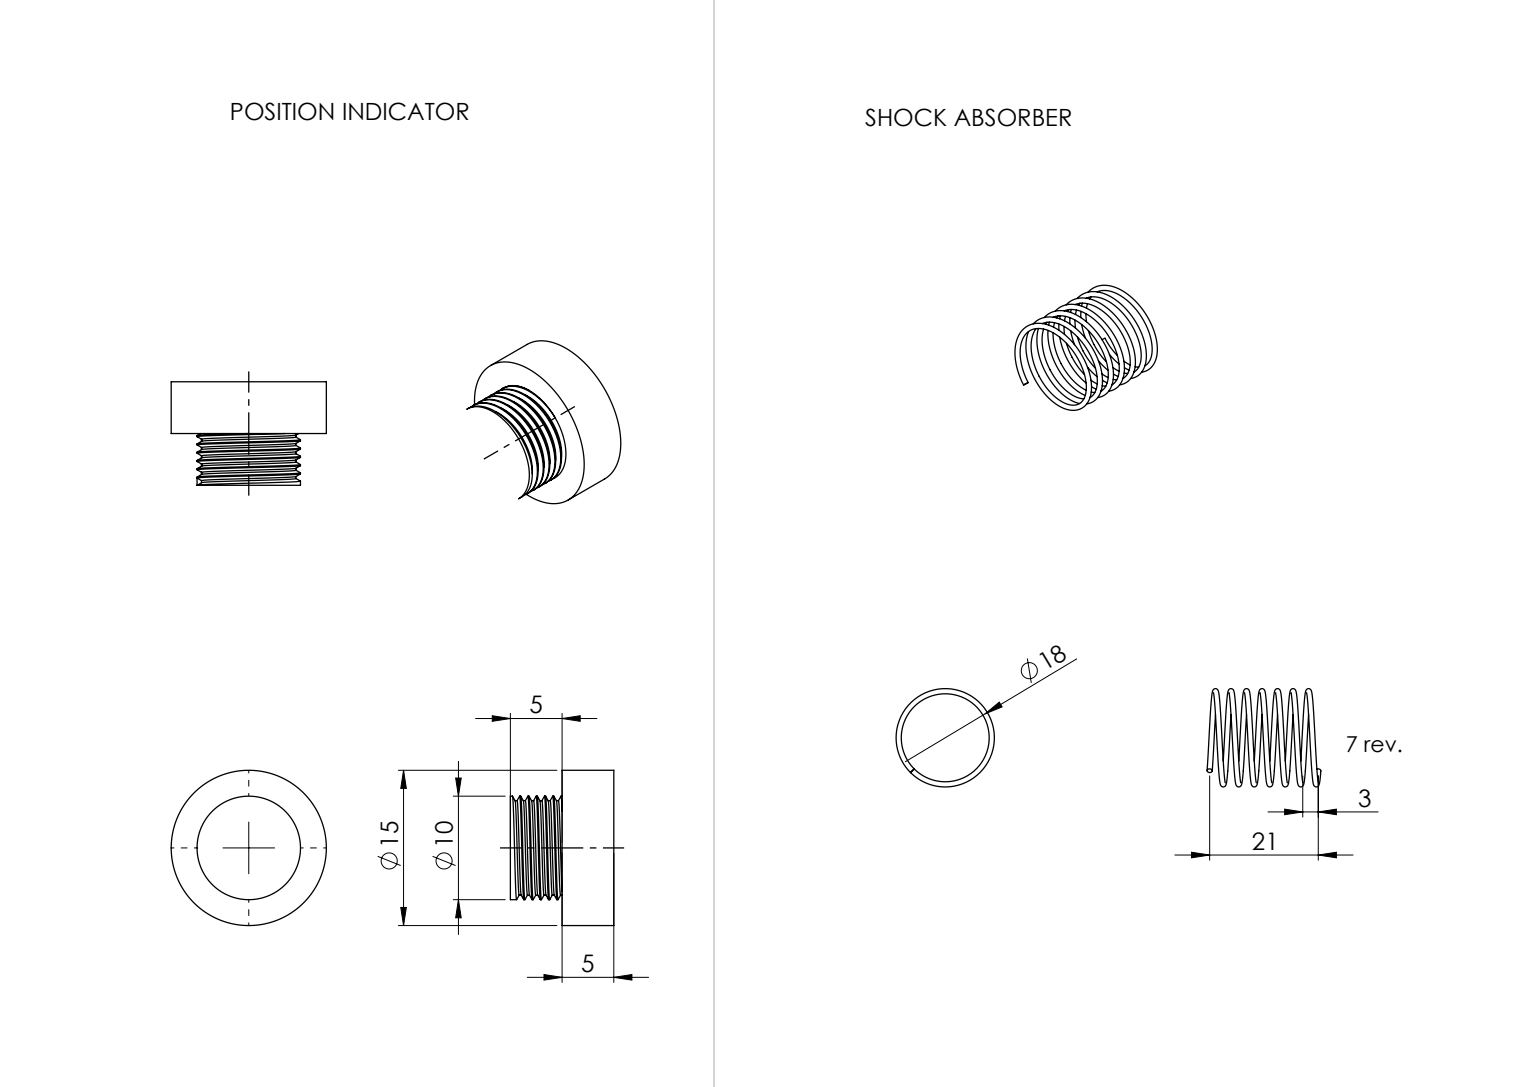
ISO-10303-21;
HEADER;
FILE_DESCRIPTION (('STEP AP214'),
    '1' );
FILE_NAME ('shock absorber.step',
    '2026-09-29T11:11:29',
    ( '' ),
    ( '' ),
    'SwSTEP 2.0',
    'SolidWorks 2026',
    '' );
FILE_SCHEMA (( 'AUTOMOTIVE_DESIGN' ));
ENDSEC;

DATA;
#6=CARTESIAN_POINT ( 'NONE',  ( -39.38303923565386100, -41.70000000000000995, -1.486127417882099788 ) ) ;
#7=CARTESIAN_POINT ( 'NONE',  ( -22.03669253526174998, -31.34999999999999787, 4.057507815433014642 ) ) ;
#11=CARTESIAN_POINT ( 'NONE',  ( -21.55948914237271907, -43.89859572486944472, -4.360112732550413206 ) ) ;
#17=CARTESIAN_POINT ( 'NONE',  ( -28.67030704715798350, -46.80000000000001137, 8.395350895058669494 ) ) ;
#18=CARTESIAN_POINT ( 'NONE',  ( -31.50758917197619979, -41.94859572486944188, 9.874625247442176956 ) ) ;
#19=CARTESIAN_POINT ( 'NONE',  ( -22.89739904353894318, -38.75140427513058228, -7.023824353025938549 ) ) ;
#23=CARTESIAN_POINT ( 'NONE',  ( -21.12512167993187973, -48.35140427513057659, 4.584493831696868860 ) ) ;
#30=CARTESIAN_POINT ( 'NONE',  ( -22.03669253526174998, -49.35000000000000853, 4.057507815433014642 ) ) ;
#31=CARTESIAN_POINT ( 'NONE',  ( -23.28248557872775137, -37.50000000000000711, 6.717514421272141156 ) ) ;
#36=CARTESIAN_POINT ( 'NONE',  ( -34.53486167607238144, -42.15000000000001279, -8.900167166472096270 ) ) ;
#40=CARTESIAN_POINT ( 'NONE',  ( -28.54686042191934092, -41.45140427513058512, -8.818680382772479120 ) ) ;
#43=CARTESIAN_POINT ( 'NONE',  ( -23.68028341417693738, -42.75000000000000711, -6.319716585823200283 ) ) ;
#50=CARTESIAN_POINT ( 'NONE',  ( -21.09983283352784156, -49.35000000000000853, 4.534861676072186043 ) ) ;
#51=CARTESIAN_POINT ( 'NONE',  ( -21.17260567462091458, -31.05000000000000782, -1.398121909749242331 ) ) ;
#55=CARTESIAN_POINT ( 'NONE',  ( -23.24502507771338600, -44.49859572486944614, 6.680053920257780220 ) ) ;
#57=CARTESIAN_POINT ( 'NONE',  ( -21.09983283352783801, -34.35000000000000853, 4.534861676072186043 ) ) ;
#61=CARTESIAN_POINT ( 'NONE',  ( -34.10713997105786888, -31.14859572486944828, -7.938018618334151455 ) ) ;
#62=CARTESIAN_POINT ( 'NONE',  ( -25.73429323749904185, -40.59859572486944757, -8.488613101951701267 ) ) ;
#63=CARTESIAN_POINT ( 'NONE',  ( -31.61762450863942320, -45.95140427513058512, 9.857197362228843573 ) ) ;
#64=ORIENTED_EDGE ( 'NONE', *, *, #7792, .F. ) ;
#66=CARTESIAN_POINT ( 'NONE',  ( -22.89739904353894318, -41.75140427513057517, -7.023824353025938549 ) ) ;
#72=CARTESIAN_POINT ( 'NONE',  ( -31.38201786482021305, -34.29859572486943620, -8.387063443159975762 ) ) ;
#73=CARTESIAN_POINT ( 'NONE',  ( -39.86591130483550671, -32.55000000000000426, 1.562606840307984468 ) ) ;
#84=CARTESIAN_POINT ( 'NONE',  ( -31.45313957808072303, -39.95140427513058512, 8.818680382772479120 ) ) ;
#91=CARTESIAN_POINT ( 'NONE',  ( -22.03669253526174998, -43.35000000000000853, 4.057507815433014642 ) ) ;
#97=CARTESIAN_POINT ( 'NONE',  ( -25.46513832392765408, -46.65000000000001279, 8.900167166472096270 ) ) ;
#98=CARTESIAN_POINT ( 'NONE',  ( -34.05750781543318340, -33.15000000000001279, -7.963307464738195840 ) ) ;
#103=CARTESIAN_POINT ( 'NONE',  ( -25.73429323749904185, -43.59859572486944046, -8.488613101951701267 ) ) ;
#105=CARTESIAN_POINT ( 'NONE',  ( -23.28248557872775137, -34.50000000000000000, 6.717514421272141156 ) ) ;
#106=EDGE_LOOP ( 'NONE', ( #3791, #8082, #1167, #64 ) ) ;
#109=CARTESIAN_POINT ( 'NONE',  ( -25.94249218456686279, -46.65000000000001279, 7.963307464738195840 ) ) ;
#110=CARTESIAN_POINT ( 'NONE',  ( -31.53845232986046554, -43.29859572486943620, -9.374751783755117529 ) ) ;
#111=CARTESIAN_POINT ( 'NONE',  ( -36.68005392025794009, -41.00140427513057517, -6.754974922286504757 ) ) ;
#115=CARTESIAN_POINT ( 'NONE',  ( -23.28248557872775137, -31.50000000000000711, 6.717514421272141156 ) ) ;
#121=CARTESIAN_POINT ( 'NONE',  ( -33.85891924778610473, -50.10000000000000853, 7.573555455601171715 ) ) ;
#122=CARTESIAN_POINT ( 'NONE',  ( -25.46513832392765408, -31.65000000000000568, 8.900167166472096270 ) ) ;
#124=CARTESIAN_POINT ( 'NONE',  ( -20.13408869516453947, -46.05000000000001137, -1.562606840307983136 ) ) ;
#131=CARTESIAN_POINT ( 'NONE',  ( -38.83610826798580717, -46.55140427513058654, 1.343104241417631073 ) ) ;
#134=CARTESIAN_POINT ( 'NONE',  ( -31.32969295284206979, -48.30000000000001137, -8.395350895058669494 ) ) ;
#142=CARTESIAN_POINT ( 'NONE',  ( -25.94249218456686279, -34.64999999999998437, 7.963307464738195840 ) ) ;
#146=CARTESIAN_POINT ( 'NONE',  ( -34.58449383169706692, -46.14859572486944472, -8.874878320068054549 ) ) ;
#148=CARTESIAN_POINT ( 'NONE',  ( -20.61696076434619584, -34.20000000000000995, 1.486127417882100676 ) ) ;
#153=CARTESIAN_POINT ( 'NONE',  ( -21.59636165304264921, -38.19859572486942767, 1.277368040863740228 ) ) ;
#155=CARTESIAN_POINT ( 'NONE',  ( -21.07454398712378918, -44.34859572486944046, 4.485229520447505003 ) ) ;
#156=CARTESIAN_POINT ( 'NONE',  ( -39.37475178375516549, -43.70140427513058512, -1.538452329860249712 ) ) ;
#167=CARTESIAN_POINT ( 'NONE',  ( -38.81868038277247734, -36.54859572486943620, 1.453139578080855365 ) ) ;
#168=CARTESIAN_POINT ( 'NONE',  ( -36.71751442127229836, -30.00000000000000711, -6.717514421272142044 ) ) ;
#170=CARTESIAN_POINT ( 'NONE',  ( -25.68709025247441602, -48.60000000000000142, -8.464561979789547053 ) ) ;
#178=CARTESIAN_POINT ( 'NONE',  ( -23.64089511245930098, -44.75140427513058228, -6.280328284105564762 ) ) ;
#182=CARTESIAN_POINT ( 'NONE',  ( -23.68028341417693738, -48.75000000000000711, -6.319716585823200283 ) ) ;
#185=CARTESIAN_POINT ( 'NONE',  ( -21.60464910494133406, -37.20000000000000284, 1.329692952841886155 ) ) ;
#190=CARTESIAN_POINT ( 'NONE',  ( -38.44051085762733777, -45.39859572486944472, 4.360112732550414982 ) ) ;
#192=CARTESIAN_POINT ( 'NONE',  ( -34.31290974752564438, -32.10000000000000142, 8.464561979789547053 ) ) ;
#197=CARTESIAN_POINT ( 'NONE',  ( -26.18828373723858149, -43.59859572486944046, -7.597606577763319713 ) ) ;
#198=CARTESIAN_POINT ( 'NONE',  ( -25.68709025247441602, -30.60000000000000142, -8.464561979789547053 ) ) ;
#199=CARTESIAN_POINT ( 'NONE',  ( -38.83610826798580717, -31.55140427513057588, 1.343104241417631073 ) ) ;
#208=CARTESIAN_POINT ( 'NONE',  ( -31.38201786482021305, -46.29859572486944330, -8.387063443159975762 ) ) ;
#209=CARTESIAN_POINT ( 'NONE',  ( -34.31290974752564438, -41.10000000000000142, 8.464561979789547053 ) ) ;
#211=CARTESIAN_POINT ( 'NONE',  ( -36.71751442127229836, -45.00000000000000711, -6.717514421272142044 ) ) ;
#219=CARTESIAN_POINT ( 'NONE',  ( -37.93801861833426159, -40.85140427513057659, -4.107139971057695682 ) ) ;
#223=CARTESIAN_POINT ( 'NONE',  ( -28.67030704715798350, -46.80000000000001137, 8.395350895058669494 ) ) ;
#227=CARTESIAN_POINT ( 'NONE',  ( -23.68028341417693738, -42.75000000000001421, -6.319716585823198507 ) ) ;
#230=CARTESIAN_POINT ( 'NONE',  ( -34.53486167607238144, -33.15000000000001279, -8.900167166472096270 ) ) ;
#232=CARTESIAN_POINT ( 'NONE',  ( -21.53543802021056663, -36.90000000000000568, -4.312909747525783821 ) ) ;
#237=CARTESIAN_POINT ( 'NONE',  ( -22.45049566656107842, -40.89859572486943762, -3.906122232810846917 ) ) ;
#238=CARTESIAN_POINT ( 'NONE',  ( -21.53543802021056663, -30.90000000000000924, -4.312909747525783821 ) ) ;
#239=CARTESIAN_POINT ( 'NONE',  ( -36.68005392025794009, -47.00140427513058938, -6.754974922286504757 ) ) ;
#251=CARTESIAN_POINT ( 'NONE',  ( -37.98859631114233792, -39.84859572486944046, -4.007875659808334490 ) ) ;
#252=CARTESIAN_POINT ( 'NONE',  ( -25.46513832392765408, -43.64999999999999147, 8.900167166472096270 ) ) ;
#254=CARTESIAN_POINT ( 'NONE',  ( -34.48522952044771017, -29.15140427513058441, -8.925456012876139766 ) ) ;
#261=CARTESIAN_POINT ( 'NONE',  ( -25.94249218456686279, -34.64999999999998437, 7.963307464738195840 ) ) ;
#266=CARTESIAN_POINT ( 'NONE',  ( -36.01040764008574513, -51.00000000000000711, -6.010407640085605685 ) ) ;
#270=CARTESIAN_POINT ( 'NONE',  ( -22.42644454439892598, -36.90000000000000568, -3.858919247786222861 ) ) ;
#274=CARTESIAN_POINT ( 'NONE',  ( -37.06321265474346660, -32.25000000000000711, 7.063212654743582952 ) ) ;
#277=CARTESIAN_POINT ( 'NONE',  ( -23.28248557872775137, -43.50000000000001421, 6.717514421272141156 ) ) ;
#278=SURFACE_STYLE_FILL_AREA ( #8401 ) ;
#282=VERTEX_POINT ( 'NONE', #3656 ) ;
#283=CARTESIAN_POINT ( 'NONE',  ( -33.81171626276147890, -39.09859572486944046, 7.597606577763319713 ) ) ;
#284=CARTESIAN_POINT ( 'NONE',  ( -31.50758917197619979, -50.94859572486944899, 9.874625247442176956 ) ) ;
#285=CARTESIAN_POINT ( 'NONE',  ( -26.09387776718931917, -29.60140427513057659, -7.549504333439021941 ) ) ;
#294=CARTESIAN_POINT ( 'NONE',  ( -23.71967171589458445, -40.74859572486943904, -6.359104887540838469 ) ) ;
#295=CARTESIAN_POINT ( 'NONE',  ( -38.46456197978948666, -41.40000000000000568, 4.312909747525784709 ) ) ;
#298=CARTESIAN_POINT ( 'NONE',  ( -21.12512167993187973, -30.35140427513058015, 4.584493831696868860 ) ) ;
#306=CARTESIAN_POINT ( 'NONE',  ( -33.85891924778610473, -35.10000000000000853, 7.573555455601171715 ) ) ;
#310=CIRCLE ( 'NONE', #7910, 0.5000000000000001110 ) ;
#314=CARTESIAN_POINT ( 'NONE',  ( -38.39535089505872634, -35.70000000000000995, -1.329692952841885267 ) ) ;
#318=CARTESIAN_POINT ( 'NONE',  ( -25.46513832392765408, -37.65000000000000568, 8.900167166472096270 ) ) ;
#320=CARTESIAN_POINT ( 'NONE',  ( -37.06321265474346660, -44.25000000000000000, 7.063212654743582952 ) ) ;
#321=( NAMED_UNIT ( * ) PLANE_ANGLE_UNIT ( ) SI_UNIT ( $, .RADIAN. ) );
#324=CARTESIAN_POINT ( 'NONE',  ( -34.10713997105786888, -43.14859572486943762, -7.938018618334151455 ) ) ;
#325=CARTESIAN_POINT ( 'NONE',  ( -28.49241082802385350, -49.44859572486943478, -9.874625247442173404 ) ) ;
#326=CARTESIAN_POINT ( 'NONE',  ( -37.59760657776328685, -31.40140427513058086, 3.811716262761598362 ) ) ;
#329=CARTESIAN_POINT ( 'NONE',  ( -21.09983283352784156, -40.35000000000000142, 4.534861676072186043 ) ) ;
#334=CARTESIAN_POINT ( 'NONE',  ( -22.01140368885771892, -38.34859572486944046, 4.007875659808335378 ) ) ;
#336=CARTESIAN_POINT ( 'NONE',  ( -22.93678734525658314, -42.75000000000001421, -7.063212654743582952 ) ) ;
#338=CARTESIAN_POINT ( 'NONE',  ( -25.51477047955235378, -39.65140427513058086, 8.925456012876139766 ) ) ;
#345=CARTESIAN_POINT ( 'NONE',  ( -26.14108075221394856, -30.60000000000000142, -7.573555455601170827 ) ) ;
#352=CARTESIAN_POINT ( 'NONE',  ( -36.31971658582311591, -44.25000000000000000, 6.319716585823199395 ) ) ;
#357=CARTESIAN_POINT ( 'NONE',  ( -21.53543802021056663, -36.90000000000000568, -4.312909747525783821 ) ) ;
#359=CARTESIAN_POINT ( 'NONE',  ( -25.68709025247441602, -36.60000000000000853, -8.464561979789547053 ) ) ;
#361=CARTESIAN_POINT ( 'NONE',  ( -36.04786814110010340, -51.99859572486943193, -5.972947139071243861 ) ) ;
#362=CARTESIAN_POINT ( 'NONE',  ( -20.61696076434619584, -31.20000000000000639, 1.486127417882100676 ) ) ;
#363=CARTESIAN_POINT ( 'NONE',  ( -23.64089511245930098, -32.75140427513057517, -6.280328284105564762 ) ) ;
#367=CARTESIAN_POINT ( 'NONE',  ( -21.53543802021056663, -33.90000000000000568, -4.312909747525783821 ) ) ;
#369=CARTESIAN_POINT ( 'NONE',  ( -36.01040764008574513, -30.00000000000000711, -6.010407640085605685 ) ) ;
#374=CARTESIAN_POINT ( 'NONE',  ( -37.54950433343896776, -45.39859572486944472, 3.906122232810848249 ) ) ;
#375=CARTESIAN_POINT ( 'NONE',  ( -31.48612741788231517, -45.30000000000000426, -9.383039235653804155 ) ) ;
#377=ORIENTED_EDGE ( 'NONE', *, *, #4137, .F. ) ;
#378=CARTESIAN_POINT ( 'NONE',  ( -36.68005392025794009, -32.00140427513057517, -6.754974922286504757 ) ) ;
#386=CARTESIAN_POINT ( 'NONE',  ( -33.90612223281073057, -49.10140427513058370, 7.549504333439023718 ) ) ;
#397=CARTESIAN_POINT ( 'NONE',  ( -20.13408869516454303, -43.04999999999999716, -1.562606840307982692 ) ) ;
#399=CARTESIAN_POINT ( 'NONE',  ( -28.49241082802385350, -31.44859572486944188, -9.874625247442173404 ) ) ;
#400=CARTESIAN_POINT ( 'NONE',  ( -25.46513832392765408, -40.65000000000000568, 8.900167166472096270 ) ) ;
#401=CARTESIAN_POINT ( 'NONE',  ( -23.64089511245930098, -35.75140427513057517, -6.280328284105564762 ) ) ;
#404=CARTESIAN_POINT ( 'NONE',  ( -20.13408869516453947, -34.04999999999998295, -1.562606840307983136 ) ) ;
#411=CARTESIAN_POINT ( 'NONE',  ( -37.98859631114233792, -51.84859572486944757, -4.007875659808334490 ) ) ;
#412=CARTESIAN_POINT ( 'NONE',  ( -25.46513832392765408, -49.64999999999999147, 8.900167166472096270 ) ) ;
#415=CARTESIAN_POINT ( 'NONE',  ( -21.12512167993187973, -39.35140427513057659, 4.584493831696868860 ) ) ;
#416=CIRCLE ( 'NONE', #3111, 0.5000000000000001110 ) ;
#422=CARTESIAN_POINT ( 'NONE',  ( -22.42644454439892598, -36.90000000000000568, -3.858919247786222861 ) ) ;
#435=CARTESIAN_POINT ( 'NONE',  ( -21.09983283352783801, -46.34999999999999432, 4.534861676072186043 ) ) ;
#437=CARTESIAN_POINT ( 'NONE',  ( -38.81868038277247734, -45.54859572486944330, 1.453139578080855365 ) ) ;
#438=CARTESIAN_POINT ( 'NONE',  ( -21.53543802021056663, -36.90000000000000568, -4.312909747525783821 ) ) ;
#440=CARTESIAN_POINT ( 'NONE',  ( -37.59760657776328685, -40.40140427513058086, 3.811716262761598362 ) ) ;
#444=CARTESIAN_POINT ( 'NONE',  ( -38.92545601287626056, -36.84859572486944046, -4.485229520447501450 ) ) ;
#445=CARTESIAN_POINT ( 'NONE',  ( -31.48612741788231517, -36.30000000000000426, -9.383039235653804155 ) ) ;
#452=CARTESIAN_POINT ( 'NONE',  ( -31.38201786482021305, -49.29859572486945041, -8.387063443159975762 ) ) ;
#453=CARTESIAN_POINT ( 'NONE',  ( -21.12512167993187973, -33.35140427513057659, 4.584493831696868860 ) ) ;
#457=CARTESIAN_POINT ( 'NONE',  ( -21.51138689804841420, -35.90140427513058086, -4.265706762501151772 ) ) ;
#464=CARTESIAN_POINT ( 'NONE',  ( -37.96330746473829976, -38.85000000000001563, -4.057507815433013754 ) ) ;
#470=CARTESIAN_POINT ( 'NONE',  ( -24.02705286092866643, -33.50140427513058228, 6.047868141099968398 ) ) ;
#473=CARTESIAN_POINT ( 'NONE',  ( -23.68028341417693738, -36.75000000000000711, -6.319716585823200283 ) ) ;
#475=CARTESIAN_POINT ( 'NONE',  ( -37.06321265474346660, -47.25000000000000711, 7.063212654743582952 ) ) ;
#478=CARTESIAN_POINT ( 'NONE',  ( -26.18828373723858149, -46.59859572486944046, -7.597606577763319713 ) ) ;
#479=CARTESIAN_POINT ( 'NONE',  ( -39.86591130483550671, -38.54999999999999716, 1.562606840307984468 ) ) ;
#480=CARTESIAN_POINT ( 'NONE',  ( -33.90612223281073057, -40.10140427513057659, 7.549504333439023718 ) ) ;
#484=CARTESIAN_POINT ( 'NONE',  ( -21.55948914237271907, -40.89859572486943762, -4.360112732550413206 ) ) ;
#485=CARTESIAN_POINT ( 'NONE',  ( -38.46456197978948666, -35.40000000000000568, 4.312909747525784709 ) ) ;
#493=CARTESIAN_POINT ( 'NONE',  ( -34.26570676250101855, -33.09859572486943335, 8.488613101951703044 ) ) ;
#494=CARTESIAN_POINT ( 'NONE',  ( -28.56619749409589204, -33.80140427513056522, 9.391326687552490782 ) ) ;
#496=AXIS2_PLACEMENT_3D ( 'NONE', #718, #6149, #4079 ) ;
#499=CARTESIAN_POINT ( 'NONE',  ( -25.63988726744978663, -38.60140427513057659, -8.440510857627391061 ) ) ;
#507=CARTESIAN_POINT ( 'NONE',  ( -21.60464910494133406, -40.20000000000000995, 1.329692952841886155 ) ) ;
#513=CARTESIAN_POINT ( 'NONE',  ( -39.38303923565386100, -35.70000000000000995, -1.486127417882099788 ) ) ;
#516=CARTESIAN_POINT ( 'NONE',  ( -34.00787565980851213, -32.15140427513058086, -7.988596311142238449 ) ) ;
#519=CARTESIAN_POINT ( 'NONE',  ( -38.82739432537914581, -38.55000000000000426, 1.398121909749243663 ) ) ;
#521=CARTESIAN_POINT ( 'NONE',  ( -21.53543802021056663, -48.90000000000000568, -4.312909747525783821 ) ) ;
#524=CARTESIAN_POINT ( 'NONE',  ( -37.54950433343896776, -48.39859572486944472, 3.906122232810848249 ) ) ;
#525=CARTESIAN_POINT ( 'NONE',  ( -39.38303923565386100, -35.70000000000000995, -1.486127417882099788 ) ) ;
#526=CARTESIAN_POINT ( 'NONE',  ( -35.97294713907137975, -35.00140427513057517, -6.047868141099968398 ) ) ;
#530=CARTESIAN_POINT ( 'NONE',  ( -31.50758917197619979, -41.94859572486944188, 9.874625247442176956 ) ) ;
#531=CARTESIAN_POINT ( 'NONE',  ( -20.61696076434619584, -43.20000000000000995, 1.486127417882100676 ) ) ;
#539=CARTESIAN_POINT ( 'NONE',  ( -21.59636165304264921, -47.19859572486943478, 1.277368040863740228 ) ) ;
#540=CARTESIAN_POINT ( 'NONE',  ( -39.87462524744216807, -34.55140427513057233, 1.507589171976367215 ) ) ;
#543=CARTESIAN_POINT ( 'NONE',  ( -28.38237549136062654, -44.45140427513058512, -9.857197362228843573 ) ) ;
#551=CARTESIAN_POINT ( 'NONE',  ( -38.39535089505872634, -44.70000000000000284, -1.329692952841885267 ) ) ;
#555=CARTESIAN_POINT ( 'NONE',  ( -22.93678734525658314, -39.74999999999999289, -7.063212654743582952 ) ) ;
#559=CARTESIAN_POINT ( 'NONE',  ( -37.93801861833426159, -37.85140427513057659, -4.107139971057695682 ) ) ;
#562=CARTESIAN_POINT ( 'NONE',  ( -34.05750781543319050, -39.14999999999999858, -7.963307464738194952 ) ) ;
#565=CARTESIAN_POINT ( 'NONE',  ( -39.86591130483550671, -50.55000000000001137, 1.562606840307984690 ) ) ;
#569=CARTESIAN_POINT ( 'NONE',  ( -36.71751442127229836, -39.00000000000000711, -6.717514421272142044 ) ) ;
#570=CARTESIAN_POINT ( 'NONE',  ( -34.00787565980851213, -38.15140427513058086, -7.988596311142238449 ) ) ;
#573=CARTESIAN_POINT ( 'NONE',  ( -25.41550616830297571, -32.64859572486943762, 8.874878320068054549 ) ) ;
#574=CARTESIAN_POINT ( 'NONE',  ( -31.50758917197619979, -32.94859572486944188, 9.874625247442176956 ) ) ;
#582=CARTESIAN_POINT ( 'NONE',  ( -36.01040764008574513, -48.00000000000000711, -6.010407640085605685 ) ) ;
#583=CARTESIAN_POINT ( 'NONE',  ( -23.24502507771338600, -32.49859572486943904, 6.680053920257780220 ) ) ;
#584=CARTESIAN_POINT ( 'NONE',  ( -20.62524821624488069, -36.20140427513057091, 1.538452329860250378 ) ) ;
#588=CARTESIAN_POINT ( 'NONE',  ( -20.12537475255788522, -42.05140427513057944, -1.507589171976365439 ) ) ;
#596=CARTESIAN_POINT ( 'NONE',  ( -31.39812190974910422, -43.95000000000000284, 8.827394325379140483 ) ) ;
#601=CARTESIAN_POINT ( 'NONE',  ( -31.48612741788231517, -42.30000000000000426, -9.383039235653804155 ) ) ;
#604=CARTESIAN_POINT ( 'NONE',  ( -22.06198138166579170, -36.35140427513057659, 4.107139971057695682 ) ) ;
#609=CARTESIAN_POINT ( 'NONE',  ( -36.31971658582311591, -38.25000000000000711, 6.319716585823200283 ) ) ;
#611=CARTESIAN_POINT ( 'NONE',  ( -28.43739315969223824, -48.45000000000000284, -9.865911304835512041 ) ) ;
#616=CARTESIAN_POINT ( 'NONE',  ( -31.48612741788231517, -42.30000000000000426, -9.383039235653804155 ) ) ;
#617=CARTESIAN_POINT ( 'NONE',  ( -26.09387776718931917, -44.60140427513058370, -7.549504333439021941 ) ) ;
#621=CARTESIAN_POINT ( 'NONE',  ( -34.58449383169706692, -40.14859572486943762, -8.874878320068054549 ) ) ;
#628=CARTESIAN_POINT ( 'NONE',  ( -25.94249218456686279, -49.64999999999999147, 7.963307464738195840 ) ) ;
#630=CARTESIAN_POINT ( 'NONE',  ( -39.39132668755255651, -39.69859572486944188, -1.433802505903950308 ) ) ;
#631=CARTESIAN_POINT ( 'NONE',  ( -25.63988726744978663, -44.60140427513058370, -8.440510857627391061 ) ) ;
#635=CARTESIAN_POINT ( 'NONE',  ( -37.10260095646111012, -46.25140427513058228, 7.023824353025939438 ) ) ;
#643=CARTESIAN_POINT ( 'NONE',  ( -31.39812190974910422, -46.94999999999998863, 8.827394325379140483 ) ) ;
#649=CARTESIAN_POINT ( 'NONE',  ( -20.13408869516453947, -40.05000000000001137, -1.562606840307983136 ) ) ;
#652=CARTESIAN_POINT ( 'NONE',  ( -23.64089511245930098, -32.75140427513057517, -6.280328284105564762 ) ) ;
#657=CARTESIAN_POINT ( 'NONE',  ( -26.14108075221394856, -39.60000000000000853, -7.573555455601170827 ) ) ;
#664=CARTESIAN_POINT ( 'NONE',  ( -20.61696076434619584, -43.20000000000000995, 1.486127417882100676 ) ) ;
#665=CARTESIAN_POINT ( 'NONE',  ( -31.27736804086391942, -44.30140427513057944, -8.403638346957361449 ) ) ;
#669=CARTESIAN_POINT ( 'NONE',  ( -25.41550616830297571, -44.64859572486944472, 8.874878320068054549 ) ) ;
#675=CARTESIAN_POINT ( 'NONE',  ( -23.98959235991431171, -49.50000000000000711, 6.010407640085604797 ) ) ;
#676=( BOUNDED_CURVE ( )  B_SPLINE_CURVE ( 2, ( #4826, #8092, #6187, #2185, #3465, #6930, #895, #2098, #6231, #6802, #7424, #2049, #809, #6886, #192, #4873, #4781, #4738, #1380, #7548, #1425, #4076, #6753, #715, #3422, #4120, #1469, #6146, #148, #57, #105, #2802, #5472, #850, #4162, #6842, #1512, #2893, #2232, #4911, #7635, #3067, #8480, #8441, #359, #4291, #232, #6445, #7018, #7683, #2935, #2363, #7817, #5745, #5610, #5785, #1027, #2405, #1070, #2445, #5698, #1783, #5083, #8311, #5126, #5654, #3721, #2275, #7772, #4955, #6315, #6974, #7731, #1741, #939, #3633, #5040, #8400, #1691, #6403, #1110, #4382, #4463, #3761, #4426, #6273, #7109, #397, #3104, #7066, #277, #3677, #1600, #6357, #2979, #320, #8355, #2320, #4998, #3026, #7149, #1646, #4338, #980, #8650, #5956, #8688, #1865, #3232, #435, #6527, #2615, #5283, #7322, #7943, #475, #7857, #3153, #5203, #7989, #7898, #2525, #5330, #611, #6655, #8604, #521, #1823, #5829, #1193, #3278, #1992, #8519, #2485, #1277, #4593, #3802, #565, #3190, #1150, #3324 ),
 .UNSPECIFIED., .F., .T. ) 
 B_SPLINE_CURVE_WITH_KNOTS ( ( 3, 2, 2, 2, 2, 2, 2, 2, 2, 2, 2, 2, 2, 2, 2, 2, 2, 2, 2, 2, 2, 2, 2, 2, 2, 2, 2, 2, 2, 2, 2, 2, 2, 2, 2, 2, 2, 2, 2, 2, 2, 2, 2, 2, 2, 2, 2, 2, 2, 2, 2, 2, 2, 2, 2, 2, 2, 2, 2, 2, 2, 2, 2, 2, 2, 2, 2, 2, 2, 2, 3 ),
 ( 0.000000000000000000, 0.01428571428571428527, 0.02857142857142857054, 0.04285714285714285754, 0.05714285714285714107, 0.07142857142857142461, 0.08571428571428571508, 0.1000000000000000056, 0.1142857142857142821, 0.1285714285714285587, 0.1428571428571428492, 0.1571428571428571397, 0.1714285714285714302, 0.1857142857142857206, 0.2000000000000000111, 0.2142857142857142738, 0.2285714285714285643, 0.2428571428571428548, 0.2571428571428571175, 0.2714285714285714080, 0.2857142857142856984, 0.2999999999999999889, 0.3142857142857142794, 0.3285714285714285698, 0.3428571428571428603, 0.3571428571428571508, 0.3714285714285714413, 0.3857142857142857317, 0.4000000000000000222, 0.4142857142857143127, 0.4285714285714285476, 0.4428571428571428381, 0.4571428571428571286, 0.4714285714285714191, 0.4857142857142857095, 0.5000000000000000000, 0.5142857142857142350, 0.5285714285714285809, 0.5428571428571428159, 0.5571428571428571619, 0.5714285714285713969, 0.5857142857142857428, 0.5999999999999999778, 0.6142857142857143238, 0.6285714285714285587, 0.6428571428571429047, 0.6571428571428571397, 0.6714285714285713746, 0.6857142857142857206, 0.6999999999999999556, 0.7142857142857143016, 0.7285714285714285365, 0.7428571428571428825, 0.7571428571428571175, 0.7714285714285714635, 0.7857142857142856984, 0.8000000000000000444, 0.8142857142857142794, 0.8285714285714286254, 0.8428571428571428603, 0.8571428571428570953, 0.8714285714285714413, 0.8857142857142856762, 0.9000000000000000222, 0.9142857142857142572, 0.9285714285714286031, 0.9428571428571428381, 0.9571428571428571841, 0.9714285714285714191, 0.9857142857142857650, 1.000000000000000000 ),
 .UNSPECIFIED. ) 
 CURVE ( )  GEOMETRIC_REPRESENTATION_ITEM ( )  RATIONAL_B_SPLINE_CURVE ( ( 1.000000000000000000, 0.9510565162951535312, 1.000000000000000000, 0.9510565162951535312, 1.000000000000000000, 0.9510565162951535312, 1.000000000000000000, 0.9510565162951535312, 1.000000000000000000, 0.9510565162951535312, 1.000000000000000000, 0.9510565162951535312, 1.000000000000000000, 0.9510565162951535312, 1.000000000000000000, 0.9510565162951535312, 1.000000000000000000, 0.9510565162951535312, 1.000000000000000000, 0.9510565162951535312, 1.000000000000000000, 0.9510565162951535312, 1.000000000000000000, 0.9510565162951535312, 1.000000000000000000, 0.9510565162951535312, 1.000000000000000000, 0.9510565162951535312, 1.000000000000000000, 0.9510565162951535312, 1.000000000000000000, 0.9510565162951535312, 1.000000000000000000, 0.9510565162951535312, 1.000000000000000000, 0.9510565162951535312, 1.000000000000000000, 0.9510565162951535312, 1.000000000000000000, 0.9510565162951535312, 1.000000000000000000, 0.9510565162951535312, 1.000000000000000000, 0.9510565162951535312, 1.000000000000000000, 0.9510565162951535312, 1.000000000000000000, 0.9510565162951535312, 1.000000000000000000, 0.9510565162951535312, 1.000000000000000000, 0.9510565162951535312, 1.000000000000000000, 0.9510565162951535312, 1.000000000000000000, 0.9510565162951535312, 1.000000000000000000, 0.9510565162951535312, 1.000000000000000000, 0.9510565162951535312, 1.000000000000000000, 0.9510565162951535312, 1.000000000000000000, 0.9510565162951535312, 1.000000000000000000, 0.9510565162951535312, 1.000000000000000000, 0.9510565162951535312, 1.000000000000000000, 0.9510565162951535312, 1.000000000000000000, 0.9510565162951535312, 1.000000000000000000, 0.9510565162951535312, 1.000000000000000000, 0.9510565162951535312, 1.000000000000000000, 0.9510565162951535312, 1.000000000000000000, 0.9510565162951535312, 1.000000000000000000, 0.9510565162951535312, 1.000000000000000000, 0.9510565162951535312, 1.000000000000000000, 0.9510565162951535312, 1.000000000000000000, 0.9510565162951535312, 1.000000000000000000, 0.9510565162951535312, 1.000000000000000000, 0.9510565162951535312, 1.000000000000000000, 0.9510565162951535312, 1.000000000000000000, 0.9510565162951535312, 1.000000000000000000, 0.9510565162951535312, 1.000000000000000000, 0.9510565162951535312, 1.000000000000000000, 0.9510565162951535312, 1.000000000000000000, 0.9510565162951535312, 1.000000000000000000, 0.9510565162951535312, 1.000000000000000000, 0.9510565162951535312, 1.000000000000000000, 0.9510565162951535312, 1.000000000000000000, 0.9510565162951535312, 1.000000000000000000, 0.9510565162951535312, 1.000000000000000000, 0.9510565162951535312, 1.000000000000000000, 0.9510565162951535312, 1.000000000000000000, 0.9510565162951535312, 1.000000000000000000, 0.9510565162951535312, 1.000000000000000000, 0.9510565162951535312, 1.000000000000000000, 0.9510565162951535312, 1.000000000000000000, 0.9510565162951535312, 1.000000000000000000, 0.9510565162951535312, 1.000000000000000000, 0.9510565162951535312, 1.000000000000000000, 0.9510565162951535312, 1.000000000000000000, 0.9510565162951535312, 1.000000000000000000, 0.9510565162951535312, 1.000000000000000000, 0.9510565162951535312, 1.000000000000000000 ) ) 
 REPRESENTATION_ITEM ( '' )  );
#677=CARTESIAN_POINT ( 'NONE',  ( -36.75497492228666374, -39.99859572486943904, -6.680053920257780220 ) ) ;
#678=CARTESIAN_POINT ( 'NONE',  ( -28.38237549136062654, -44.45140427513058512, -9.857197362228843573 ) ) ;
#682=CARTESIAN_POINT ( 'NONE',  ( -20.12537475255788522, -45.05140427513057944, -1.507589171976365439 ) ) ;
#690=CARTESIAN_POINT ( 'NONE',  ( -23.71967171589458445, -34.74859572486943904, -6.359104887540838469 ) ) ;
#691=CARTESIAN_POINT ( 'NONE',  ( -23.28248557872775137, -34.50000000000000000, 6.717514421272141156 ) ) ;
#695=CARTESIAN_POINT ( 'NONE',  ( -37.06321265474346660, -44.25000000000000000, 7.063212654743582952 ) ) ;
#698=CARTESIAN_POINT ( 'NONE',  ( -35.97294713907137975, -41.00140427513057517, -6.047868141099968398 ) ) ;
#702=CARTESIAN_POINT ( 'NONE',  ( -33.85891924778610473, -44.10000000000000853, 7.573555455601171715 ) ) ;
#709=CARTESIAN_POINT ( 'NONE',  ( -20.13408869516453947, -49.04999999999999716, -1.562606840307983136 ) ) ;
#710=CARTESIAN_POINT ( 'NONE',  ( -26.09387776718931917, -47.60140427513058370, -7.549504333439021941 ) ) ;
#713=CARTESIAN_POINT ( 'NONE',  ( -39.85719736222883824, -51.54859572486944330, 1.617624508639602388 ) ) ;
#715=CARTESIAN_POINT ( 'NONE',  ( -28.43739315969223824, -33.45000000000000995, -9.865911304835512041 ) ) ;
#718=CARTESIAN_POINT ( 'NONE',  ( -36.36396103067902175, -51.00000000000000711, -6.363961030678874309 ) ) ;
#719=CARTESIAN_POINT ( 'NONE',  ( -36.31971658582311591, -50.24999999999998579, 6.319716585823199395 ) ) ;
#720=CARTESIAN_POINT ( 'NONE',  ( -21.07454398712378918, -38.34859572486944046, 4.485229520447505003 ) ) ;
#721=CARTESIAN_POINT ( 'NONE',  ( -38.87487832006816291, -37.85140427513057659, -4.584493831696867971 ) ) ;
#726=CARTESIAN_POINT ( 'NONE',  ( -38.87487832006816291, -43.85140427513058370, -4.584493831696867971 ) ) ;
#734=CARTESIAN_POINT ( 'NONE',  ( -37.96330746473829976, -50.84999999999999432, -4.057507815433013754 ) ) ;
#736=CARTESIAN_POINT ( 'NONE',  ( -39.86591130483550671, -38.54999999999999716, 1.562606840307984468 ) ) ;
#742=CARTESIAN_POINT ( 'NONE',  ( -28.51387258211773812, -43.80000000000000426, 9.383039235653802379 ) ) ;
#745=CARTESIAN_POINT ( 'NONE',  ( -22.06198138166579170, -42.35140427513057659, 4.107139971057695682 ) ) ;
#748=CARTESIAN_POINT ( 'NONE',  ( -22.42644454439892598, -45.90000000000001279, -3.858919247786222861 ) ) ;
#756=CARTESIAN_POINT ( 'NONE',  ( -31.56260684030781505, -49.95000000000000995, 9.865911304835510265 ) ) ;
#757=CARTESIAN_POINT ( 'NONE',  ( -38.83610826798580717, -49.55140427513056522, 1.343104241417631073 ) ) ;
#760=CARTESIAN_POINT ( 'NONE',  ( -31.50758917197619979, -47.94859572486943478, 9.874625247442176956 ) ) ;
#767=CARTESIAN_POINT ( 'NONE',  ( -34.10713997105786888, -34.14859572486943051, -7.938018618334151455 ) ) ;
#768=CARTESIAN_POINT ( 'NONE',  ( -39.85719736222883824, -42.54859572486944330, 1.617624508639602388 ) ) ;
#769=CARTESIAN_POINT ( 'NONE',  ( -21.51138689804841420, -38.90140427513058086, -4.265706762501151772 ) ) ;
#780=CARTESIAN_POINT ( 'NONE',  ( -22.01140368885771892, -32.34859572486942625, 4.007875659808335378 ) ) ;
#781=CARTESIAN_POINT ( 'NONE',  ( -21.53543802021056663, -33.90000000000000568, -4.312909747525783821 ) ) ;
#788=CARTESIAN_POINT ( 'NONE',  ( -20.13408869516453947, -49.04999999999999716, -1.562606840307983136 ) ) ;
#791=CARTESIAN_POINT ( 'NONE',  ( -38.38706344316003793, -40.70140427513058512, -1.382017864820032083 ) ) ;
#795=CARTESIAN_POINT ( 'NONE',  ( -37.57355545560112375, -47.40000000000001279, 3.858919247786223305 ) ) ;
#802=CARTESIAN_POINT ( 'NONE',  ( -31.56260684030781505, -43.95000000000000284, 9.865911304835510265 ) ) ;
#804=CARTESIAN_POINT ( 'NONE',  ( -23.64089511245930098, -44.75140427513058228, -6.280328284105564762 ) ) ;
#807=CARTESIAN_POINT ( 'NONE',  ( -23.24502507771338600, -50.49859572486944614, 6.680053920257780220 ) ) ;
#809=CARTESIAN_POINT ( 'NONE',  ( -28.51387258211773812, -31.80000000000000782, 9.383039235653802379 ) ) ;
#813=CARTESIAN_POINT ( 'NONE',  ( -22.01140368885771892, -41.34859572486944757, 4.007875659808335378 ) ) ;
#814=CARTESIAN_POINT ( 'NONE',  ( -20.60867331244750034, -38.19859572486942767, 1.433802505903951419 ) ) ;
#815=CARTESIAN_POINT ( 'NONE',  ( -39.37475178375516549, -40.70140427513058512, -1.538452329860249712 ) ) ;
#825=CARTESIAN_POINT ( 'NONE',  ( -37.98859631114233792, -33.84859572486942625, -4.007875659808334490 ) ) ;
#826=CARTESIAN_POINT ( 'NONE',  ( -28.43739315969223824, -36.45000000000000284, -9.865911304835512041 ) ) ;
#828=CARTESIAN_POINT ( 'NONE',  ( -31.48612741788231517, -48.30000000000001137, -9.383039235653804155 ) ) ;
#833=CARTESIAN_POINT ( 'NONE',  ( -33.90612223281073057, -43.10140427513058370, 7.549504333439023718 ) ) ;
#837=CARTESIAN_POINT ( 'NONE',  ( -34.05750781543319050, -48.15000000000001279, -7.963307464738194952 ) ) ;
#841=( NAMED_UNIT ( * ) PLANE_ANGLE_UNIT ( ) SI_UNIT ( $, .RADIAN. ) );
#843=CARTESIAN_POINT ( 'NONE',  ( -36.31971658582311591, -41.25000000000000711, 6.319716585823199395 ) ) ;
#847=CARTESIAN_POINT ( 'NONE',  ( -38.44051085762733777, -42.39859572486944472, 4.360112732550414982 ) ) ;
#850=CARTESIAN_POINT ( 'NONE',  ( -31.56260684030781505, -34.95000000000000995, 9.865911304835508489 ) ) ;
#854=CARTESIAN_POINT ( 'NONE',  ( -37.98859631114233792, -39.84859572486944046, -4.007875659808334490 ) ) ;
#855=CARTESIAN_POINT ( 'NONE',  ( -37.02382435302582309, -51.24859572486943193, 7.102600956461226467 ) ) ;
#856=CARTESIAN_POINT ( 'NONE',  ( -34.00787565980851213, -29.15140427513058441, -7.988596311142238449 ) ) ;
#866=CARTESIAN_POINT ( 'NONE',  ( -36.01040764008574513, -51.00000000000000711, -6.010407640085605685 ) ) ;
#867=CARTESIAN_POINT ( 'NONE',  ( -38.46456197978948666, -47.40000000000001279, 4.312909747525784709 ) ) ;
#869=CARTESIAN_POINT ( 'NONE',  ( -21.53543802021056663, -45.90000000000001279, -4.312909747525783821 ) ) ;
#877=CARTESIAN_POINT ( 'NONE',  ( -34.00787565980851213, -47.15140427513058086, -7.988596311142238449 ) ) ;
#882=CARTESIAN_POINT ( 'NONE',  ( -31.39812190974910422, -46.94999999999999574, 8.827394325379140483 ) ) ;
#887=CARTESIAN_POINT ( 'NONE',  ( -22.42644454439892598, -33.90000000000000568, -3.858919247786222861 ) ) ;
#892=CARTESIAN_POINT ( 'NONE',  ( -25.46513832392765408, -31.65000000000000568, 8.900167166472096270 ) ) ;
#895=CARTESIAN_POINT ( 'NONE',  ( -21.53543802021056663, -30.90000000000000924, -4.312909747525783821 ) ) ;
#900=CARTESIAN_POINT ( 'NONE',  ( -38.40363834695740053, -36.69859572486944188, -1.277368040863739118 ) ) ;
#901=CARTESIAN_POINT ( 'NONE',  ( -25.41550616830297571, -44.64859572486944472, 8.874878320068054549 ) ) ;
#902=CARTESIAN_POINT ( 'NONE',  ( -22.06198138166579170, -33.35140427513057659, 4.107139971057695682 ) ) ;
#913=CARTESIAN_POINT ( 'NONE',  ( -21.59636165304264921, -38.19859572486942767, 1.277368040863740228 ) ) ;
#914=CARTESIAN_POINT ( 'NONE',  ( -39.38303923565386100, -41.70000000000000995, -1.486127417882099788 ) ) ;
#917=CARTESIAN_POINT ( 'NONE',  ( -39.86591130483550671, -44.55000000000001137, 1.562606840307984468 ) ) ;
#924=CARTESIAN_POINT ( 'NONE',  ( -25.94249218456686279, -31.65000000000000568, 7.963307464738195840 ) ) ;
#926=EDGE_CURVE ( 'NONE', #4270, #282, #310, .T. ) ;
#934=CARTESIAN_POINT ( 'NONE',  ( -37.96330746473829976, -35.84999999999998721, -4.057507815433013754 ) ) ;
#937=CARTESIAN_POINT ( 'NONE',  ( -36.71751442127229836, -36.00000000000000711, -6.717514421272142044 ) ) ;
#939=CARTESIAN_POINT ( 'NONE',  ( -34.31290974752564438, -41.10000000000000142, 8.464561979789547053 ) ) ;
#943=CARTESIAN_POINT ( 'NONE',  ( -31.38201786482021305, -37.29859572486943620, -8.387063443159975762 ) ) ;
#944=CARTESIAN_POINT ( 'NONE',  ( -22.97617564697422665, -46.74859572486943904, -7.102600956461224690 ) ) ;
#945=CARTESIAN_POINT ( 'NONE',  ( -28.54686042191934092, -29.45140427513057801, -8.818680382772479120 ) ) ;
#956=CARTESIAN_POINT ( 'NONE',  ( -28.65689575858256077, -40.44859572486944188, -8.836108267985801845 ) ) ;
#957=CARTESIAN_POINT ( 'NONE',  ( -25.46513832392765408, -46.65000000000001279, 8.900167166472096270 ) ) ;
#960=CARTESIAN_POINT ( 'NONE',  ( -20.12537475255788522, -30.05140427513057944, -1.507589171976365439 ) ) ;
#968=CARTESIAN_POINT ( 'NONE',  ( -31.45313957808072303, -48.95140427513057091, 8.818680382772479120 ) ) ;
#974=( LENGTH_UNIT ( ) NAMED_UNIT ( * ) SI_UNIT ( .MILLI., .METRE. ) );
#975=CARTESIAN_POINT ( 'NONE',  ( -37.96330746473829976, -38.85000000000001563, -4.057507815433013754 ) ) ;
#977=CARTESIAN_POINT ( 'NONE',  ( -36.01040764008574513, -30.00000000000000711, -6.010407640085605685 ) ) ;
#978=CARTESIAN_POINT ( 'NONE',  ( -28.43739315969223824, -30.44999999999999574, -9.865911304835512041 ) ) ;
#980=CARTESIAN_POINT ( 'NONE',  ( -28.43739315969223824, -45.45000000000000284, -9.865911304835512041 ) ) ;
#984=CARTESIAN_POINT ( 'NONE',  ( -31.34310424141748896, -35.94859572486944188, 8.836108267985801845 ) ) ;
#985=CARTESIAN_POINT ( 'NONE',  ( -39.85719736222883824, -45.54859572486944330, 1.617624508639602388 ) ) ;
#986=CARTESIAN_POINT ( 'NONE',  ( -25.63988726744978663, -47.60140427513058370, -8.440510857627391061 ) ) ;
#996=CARTESIAN_POINT ( 'NONE',  ( -38.40363834695740053, -42.69859572486944188, -1.277368040863739118 ) ) ;
#997=CARTESIAN_POINT ( 'NONE',  ( -20.61696076434619584, -43.20000000000000995, 1.486127417882100676 ) ) ;
#1000=CARTESIAN_POINT ( 'NONE',  ( -36.68005392025794009, -38.00140427513057517, -6.754974922286504757 ) ) ;
#1010=CARTESIAN_POINT ( 'NONE',  ( -37.57355545560112375, -35.40000000000000568, 3.858919247786223305 ) ) ;
#1020=CARTESIAN_POINT ( 'NONE',  ( -25.94249218456686279, -43.64999999999999147, 7.963307464738195840 ) ) ;
#1025=CARTESIAN_POINT ( 'NONE',  ( -31.56260684030781505, -37.94999999999998153, 9.865911304835510265 ) ) ;
#1027=CARTESIAN_POINT ( 'NONE',  ( -38.46456197978948666, -38.40000000000000568, 4.312909747525784709 ) ) ;
#1032=CARTESIAN_POINT ( 'NONE',  ( -21.59636165304264921, -50.19859572486944188, 1.277368040863740228 ) ) ;
#1033=CARTESIAN_POINT ( 'NONE',  ( -23.24502507771338600, -47.49859572486944614, 6.680053920257780220 ) ) ;
#1034=CARTESIAN_POINT ( 'NONE',  ( -33.90612223281073057, -31.10140427513058370, 7.549504333439023718 ) ) ;
#1037=CARTESIAN_POINT ( 'NONE',  ( -38.90016716647221529, -38.85000000000001563, -4.534861676072185155 ) ) ;
#1038=PLANE ( 'NONE',  #1408 ) ;
#1043=CARTESIAN_POINT ( 'NONE',  ( -34.10713997105786888, -37.14859572486943762, -7.938018618334151455 ) ) ;
#1045=CARTESIAN_POINT ( 'NONE',  ( -28.51387258211773812, -43.80000000000000426, 9.383039235653802379 ) ) ;
#1047=CARTESIAN_POINT ( 'NONE',  ( -36.68005392025794009, -35.00140427513057517, -6.754974922286504757 ) ) ;
#1054=CARTESIAN_POINT ( 'NONE',  ( -22.03669253526174998, -37.35000000000000853, 4.057507815433014642 ) ) ;
#1068=CARTESIAN_POINT ( 'NONE',  ( -34.53486167607238144, -39.14999999999999147, -8.900167166472096270 ) ) ;
#1070=CARTESIAN_POINT ( 'NONE',  ( -39.38303923565386100, -38.70000000000000284, -1.486127417882099788 ) ) ;
#1073=CARTESIAN_POINT ( 'NONE',  ( -25.89286002894218086, -50.64859572486944472, 7.938018618334153231 ) ) ;
#1074=CARTESIAN_POINT ( 'NONE',  ( -36.71751442127229836, -36.00000000000000711, -6.717514421272142044 ) ) ;
#1075=CARTESIAN_POINT ( 'NONE',  ( -21.16389173201424612, -39.05140427513057944, -1.343104241417630185 ) ) ;
#1079=CARTESIAN_POINT ( 'NONE',  ( -38.90016716647221529, -35.84999999999998721, -4.534861676072185155 ) ) ;
#1085=CARTESIAN_POINT ( 'NONE',  ( -36.28032828410546529, -45.24859572486943904, 6.359104887540839357 ) ) ;
#1086=CARTESIAN_POINT ( 'NONE',  ( -39.86591130483550671, -50.55000000000001137, 1.562606840307984468 ) ) ;
#1090=CARTESIAN_POINT ( 'NONE',  ( -25.63988726744978663, -35.60140427513057659, -8.440510857627391061 ) ) ;
#1099=CARTESIAN_POINT ( 'NONE',  ( -38.38706344316003793, -49.70140427513058512, -1.382017864820032083 ) ) ;
#1102=CARTESIAN_POINT ( 'NONE',  ( -38.82739432537914581, -50.55000000000001137, 1.398121909749243663 ) ) ;
#1106=FACE_OUTER_BOUND ( 'NONE', #106, .T. ) ;
#1110=CARTESIAN_POINT ( 'NONE',  ( -36.71751442127229836, -42.00000000000000711, -6.717514421272142044 ) ) ;
#1111=( NAMED_UNIT ( * ) SI_UNIT ( $, .STERADIAN. ) SOLID_ANGLE_UNIT ( ) );
#1113=CARTESIAN_POINT ( 'NONE',  ( -38.40363834695740053, -45.69859572486943478, -1.277368040863739118 ) ) ;
#1114=CARTESIAN_POINT ( 'NONE',  ( -37.06321265474346660, -41.25000000000000711, 7.063212654743582952 ) ) ;
#1115=CARTESIAN_POINT ( 'NONE',  ( -37.59760657776328685, -43.40140427513058796, 3.811716262761598362 ) ) ;
#1118=CARTESIAN_POINT ( 'NONE',  ( -25.73429323749904185, -40.59859572486944757, -8.488613101951701267 ) ) ;
#1119=CARTESIAN_POINT ( 'NONE',  ( -37.06321265474346660, -35.24999999999998579, 7.063212654743582952 ) ) ;
#1126=CARTESIAN_POINT ( 'NONE',  ( -37.54950433343896776, -48.39859572486944472, 3.906122232810848249 ) ) ;
#1127=CARTESIAN_POINT ( 'NONE',  ( -20.12537475255788522, -33.05140427513057233, -1.507589171976365439 ) ) ;
#1129=CARTESIAN_POINT ( 'NONE',  ( -25.51477047955235378, -33.65140427513057375, 8.925456012876139766 ) ) ;
#1138=CARTESIAN_POINT ( 'NONE',  ( -36.31971658582311591, -41.25000000000000711, 6.319716585823199395 ) ) ;
#1143=CARTESIAN_POINT ( 'NONE',  ( -28.72263195913613387, -30.80140427513057233, 8.403638346957361449 ) ) ;
#1144=CARTESIAN_POINT ( 'NONE',  ( -22.42644454439892598, -39.90000000000000568, -3.858919247786222861 ) ) ;
#1147=CARTESIAN_POINT ( 'NONE',  ( -36.31971658582311591, -32.25000000000000711, 6.319716585823200283 ) ) ;
#1150=CARTESIAN_POINT ( 'NONE',  ( -38.90016716647221529, -50.85000000000000142, -4.534861676072185155 ) ) ;
#1153=CARTESIAN_POINT ( 'NONE',  ( -28.61798213517984024, -44.79859572486943620, 8.387063443159973986 ) ) ;
#1154=CARTESIAN_POINT ( 'NONE',  ( -25.68709025247441602, -36.60000000000000853, -8.464561979789547053 ) ) ;
#1156=CARTESIAN_POINT ( 'NONE',  ( -21.61293655684001536, -36.20140427513057091, 1.382017864820032971 ) ) ;
#1161=CARTESIAN_POINT ( 'NONE',  ( -28.49241082802385350, -37.44859572486943478, -9.874625247442173404 ) ) ;
#1162=CARTESIAN_POINT ( 'NONE',  ( -37.06321265474346660, -32.25000000000000711, 7.063212654743582952 ) ) ;
#1167=ORIENTED_EDGE ( 'NONE', *, *, #3403, .T. ) ;
#1169=CARTESIAN_POINT ( 'NONE',  ( -38.81868038277247734, -48.54859572486944330, 1.453139578080855365 ) ) ;
#1170=CARTESIAN_POINT ( 'NONE',  ( -20.62524821624488069, -33.20140427513057091, 1.538452329860250378 ) ) ;
#1175=CARTESIAN_POINT ( 'NONE',  ( -39.87462524744216807, -37.55140427513057944, 1.507589171976367215 ) ) ;
#1184=CARTESIAN_POINT ( 'NONE',  ( -36.31971658582311591, -47.25000000000000711, 6.319716585823199395 ) ) ;
#1188=CARTESIAN_POINT ( 'NONE',  ( -31.45313957808072303, -36.95140427513057801, 8.818680382772479120 ) ) ;
#1191=CARTESIAN_POINT ( 'NONE',  ( -36.31971658582311591, -35.25000000000000000, 6.319716585823200283 ) ) ;
#1193=CARTESIAN_POINT ( 'NONE',  ( -21.09983283352783801, -49.35000000000000853, 4.534861676072186043 ) ) ;
#1196=CARTESIAN_POINT ( 'NONE',  ( -36.28032828410546529, -45.24859572486943904, 6.359104887540839357 ) ) ;
#1197=CARTESIAN_POINT ( 'NONE',  ( -25.46513832392765408, -37.65000000000000568, 8.900167166472096270 ) ) ;
#1198=CARTESIAN_POINT ( 'NONE',  ( -37.93801861833426159, -43.85140427513058370, -4.107139971057695682 ) ) ;
#1203=CARTESIAN_POINT ( 'NONE',  ( -38.92545601287626056, -39.84859572486944046, -4.485229520447501450 ) ) ;
#1204=CARTESIAN_POINT ( 'NONE',  ( -36.71751442127229836, -39.00000000000000711, -6.717514421272142044 ) ) ;
#1211=CARTESIAN_POINT ( 'NONE',  ( -21.18131961722757595, -50.04859572486944330, -1.453139578080854699 ) ) ;
#1212=CARTESIAN_POINT ( 'NONE',  ( -38.90016716647221529, -50.84999999999999432, -4.534861676072185155 ) ) ;
#1216=CARTESIAN_POINT ( 'NONE',  ( -39.37475178375516549, -40.70140427513058512, -1.538452329860249712 ) ) ;
#1223=CARTESIAN_POINT ( 'NONE',  ( -22.42644454439892598, -42.90000000000000568, -3.858919247786222861 ) ) ;
#1228=CARTESIAN_POINT ( 'NONE',  ( -20.61696076434619584, -46.20000000000000284, 1.486127417882100676 ) ) ;
#1231=CARTESIAN_POINT ( 'NONE',  ( -38.38706344316003793, -37.70140427513057091, -1.382017864820032083 ) ) ;
#1234=CARTESIAN_POINT ( 'NONE',  ( -23.98959235991431171, -34.50000000000000000, 6.010407640085604797 ) ) ;
#1240=CARTESIAN_POINT ( 'NONE',  ( -21.09983283352784156, -40.35000000000000142, 4.534861676072186043 ) ) ;
#1241=CARTESIAN_POINT ( 'NONE',  ( -37.93801861833426159, -34.85140427513057659, -4.107139971057695682 ) ) ;
#1244=CARTESIAN_POINT ( 'NONE',  ( -22.97617564697422665, -37.74859572486943904, -7.102600956461224690 ) ) ;
#1251=CARTESIAN_POINT ( 'NONE',  ( -36.04786814110010340, -48.99859572486944614, -5.972947139071243861 ) ) ;
#1252=CARTESIAN_POINT ( 'NONE',  ( -28.38237549136062654, -35.45140427513057801, -9.857197362228843573 ) ) ;
#1255=CARTESIAN_POINT ( 'NONE',  ( -31.61762450863942320, -45.95140427513058512, 9.857197362228843573 ) ) ;
#1261=CARTESIAN_POINT ( 'NONE',  ( -31.32969295284206979, -39.30000000000001137, -8.395350895058669494 ) ) ;
#1267=CARTESIAN_POINT ( 'NONE',  ( -25.46513832392765408, -46.65000000000001279, 8.900167166472096270 ) ) ;
#1270=CARTESIAN_POINT ( 'NONE',  ( -38.38706344316003793, -34.70140427513057091, -1.382017864820032083 ) ) ;
#1273=CARTESIAN_POINT ( 'NONE',  ( -23.98959235991431171, -37.50000000000000711, 6.010407640085604797 ) ) ;
#1277=CARTESIAN_POINT ( 'NONE',  ( -34.31290974752564438, -50.10000000000000853, 8.464561979789547053 ) ) ;
#1280=CARTESIAN_POINT ( 'NONE',  ( -21.53543802021056663, -42.90000000000000568, -4.312909747525783821 ) ) ;
#1281=CARTESIAN_POINT ( 'NONE',  ( -23.68028341417693738, -30.75000000000000000, -6.319716585823198507 ) ) ;
#1285=CARTESIAN_POINT ( 'NONE',  ( -38.44051085762733777, -33.39859572486943762, 4.360112732550414982 ) ) ;
#1292=CARTESIAN_POINT ( 'NONE',  ( -22.42644454439892598, -45.90000000000001279, -3.858919247786222861 ) ) ;
#1294=CARTESIAN_POINT ( 'NONE',  ( -21.07454398712378918, -35.34859572486944046, 4.485229520447505003 ) ) ;
#1295=CARTESIAN_POINT ( 'NONE',  ( -23.31994607974211675, -42.50140427513057517, 6.754974922286503869 ) ) ;
#1298=CARTESIAN_POINT ( 'NONE',  ( -31.61762450863942320, -42.95140427513058512, 9.857197362228843573 ) ) ;
#1306=CARTESIAN_POINT ( 'NONE',  ( -28.67030704715798350, -46.80000000000001137, 8.395350895058669494 ) ) ;
#1312=CARTESIAN_POINT ( 'NONE',  ( -31.56260684030781505, -46.94999999999998863, 9.865911304835510265 ) ) ;
#1315=CARTESIAN_POINT ( 'NONE',  ( -28.72263195913613387, -33.80140427513056522, 8.403638346957361449 ) ) ;
#1319=CARTESIAN_POINT ( 'NONE',  ( -36.01040764008574513, -39.00000000000000711, -6.010407640085605685 ) ) ;
#1325=CARTESIAN_POINT ( 'NONE',  ( -20.13408869516453947, -46.05000000000001137, -1.562606840307983136 ) ) ;
#1326=CARTESIAN_POINT ( 'NONE',  ( -38.82739432537914581, -32.55000000000000426, 1.398121909749243441 ) ) ;
#1329=CARTESIAN_POINT ( 'NONE',  ( -38.92545601287626056, -42.84859572486944046, -4.485229520447501450 ) ) ;
#1338=CARTESIAN_POINT ( 'NONE',  ( -36.31971658582311591, -47.25000000000000711, 6.319716585823199395 ) ) ;
#1339=CARTESIAN_POINT ( 'NONE',  ( -20.14280263777121149, -35.04859572486943620, -1.617624508639600833 ) ) ;
#1340=CARTESIAN_POINT ( 'NONE',  ( -31.61762450863942320, -42.95140427513058512, 9.857197362228843573 ) ) ;
#1343=CARTESIAN_POINT ( 'NONE',  ( -28.56619749409589204, -42.80140427513057944, 9.391326687552490782 ) ) ;
#1351=CARTESIAN_POINT ( 'NONE',  ( -36.31971658582311591, -50.24999999999998579, 6.319716585823199395 ) ) ;
#1352=CARTESIAN_POINT ( 'NONE',  ( -39.38303923565386100, -35.70000000000000995, -1.486127417882099788 ) ) ;
#1357=CARTESIAN_POINT ( 'NONE',  ( -25.68709025247441602, -42.60000000000000853, -8.464561979789547053 ) ) ;
#1360=CARTESIAN_POINT ( 'NONE',  ( -21.16389173201424612, -45.05140427513057944, -1.343104241417630185 ) ) ;
#1366=CARTESIAN_POINT ( 'NONE',  ( -31.32969295284206979, -42.30000000000000426, -8.395350895058669494 ) ) ;
#1373=CARTESIAN_POINT ( 'NONE',  ( -25.68709025247441602, -48.60000000000000142, -8.464561979789547053 ) ) ;
#1374=CARTESIAN_POINT ( 'NONE',  ( -34.00787565980851213, -47.15140427513058086, -7.988596311142238449 ) ) ;
#1377=CARTESIAN_POINT ( 'NONE',  ( -22.97617564697422665, -43.74859572486943904, -7.102600956461224690 ) ) ;
#1380=CARTESIAN_POINT ( 'NONE',  ( -39.38303923565386100, -32.70000000000000995, -1.486127417882099788 ) ) ;
#1384=CARTESIAN_POINT ( 'NONE',  ( -31.32969295284206979, -48.30000000000001137, -8.395350895058669494 ) ) ;
#1385=CARTESIAN_POINT ( 'NONE',  ( -21.55948914237271907, -34.89859572486943762, -4.360112732550413206 ) ) ;
#1386=CARTESIAN_POINT ( 'NONE',  ( -36.68005392025794009, -38.00140427513057517, -6.754974922286504757 ) ) ;
#1390=CARTESIAN_POINT ( 'NONE',  ( -20.62524821624488069, -42.20140427513058512, 1.538452329860250378 ) ) ;
#1398=CARTESIAN_POINT ( 'NONE',  ( -38.82739432537914581, -50.55000000000001137, 1.398121909749243441 ) ) ;
#1399=CARTESIAN_POINT ( 'NONE',  ( -22.93678734525658314, -33.75000000000001421, -7.063212654743582952 ) ) ;
#1404=CARTESIAN_POINT ( 'NONE',  ( -25.68709025247441602, -45.60000000000000853, -8.464561979789547053 ) ) ;
#1407=CARTESIAN_POINT ( 'NONE',  ( -22.40239342223677355, -38.90140427513058086, -3.811716262761597473 ) ) ;
#1408=AXIS2_PLACEMENT_3D ( 'NONE', #5176, #3731, #6412 ) ;
#1410=CARTESIAN_POINT ( 'NONE',  ( -31.32969295284206979, -45.30000000000000426, -8.395350895058669494 ) ) ;
#1417=CARTESIAN_POINT ( 'NONE',  ( -23.28248557872775137, -49.50000000000000711, 6.717514421272141156 ) ) ;
#1419=CARTESIAN_POINT ( 'NONE',  ( -31.45313957808072303, -45.95140427513058512, 8.818680382772479120 ) ) ;
#1423=CARTESIAN_POINT ( 'NONE',  ( -31.50758917197619979, -50.94859572486944899, 9.874625247442176956 ) ) ;
#1425=CARTESIAN_POINT ( 'NONE',  ( -36.71751442127229836, -33.00000000000000711, -6.717514421272142044 ) ) ;
#1429=CARTESIAN_POINT ( 'NONE',  ( -38.39535089505872634, -50.70000000000000995, -1.329692952841885267 ) ) ;
#1430=CARTESIAN_POINT ( 'NONE',  ( -31.50758917197619979, -35.94859572486944188, 9.874625247442176956 ) ) ;
#1431=CARTESIAN_POINT ( 'NONE',  ( -25.51477047955235378, -39.65140427513058086, 8.925456012876139766 ) ) ;
#1445=CARTESIAN_POINT ( 'NONE',  ( -22.42644454439892598, -48.90000000000000568, -3.858919247786222861 ) ) ;
#1446=CARTESIAN_POINT ( 'NONE',  ( -28.43739315969223824, -39.45000000000000995, -9.865911304835512041 ) ) ;
#1456=CARTESIAN_POINT ( 'NONE',  ( -28.72263195913613387, -39.80140427513057944, 8.403638346957361449 ) ) ;
#1458=CARTESIAN_POINT ( 'NONE',  ( -37.96330746473829976, -44.85000000000000853, -4.057507815433013754 ) ) ;
#1462=CARTESIAN_POINT ( 'NONE',  ( -39.38303923565386100, -50.70000000000000995, -1.486127417882099788 ) ) ;
#1463=CARTESIAN_POINT ( 'NONE',  ( -37.59760657776328685, -49.40140427513058086, 3.811716262761598362 ) ) ;
#1467=CARTESIAN_POINT ( 'NONE',  ( -21.55948914237271907, -49.89859572486943762, -4.360112732550413206 ) ) ;
#1469=CARTESIAN_POINT ( 'NONE',  ( -21.53543802021056663, -33.90000000000000568, -4.312909747525783821 ) ) ;
#1473=CARTESIAN_POINT ( 'NONE',  ( -36.28032828410546529, -33.24859572486943193, 6.359104887540839357 ) ) ;
#1474=CARTESIAN_POINT ( 'NONE',  ( -21.55948914237271907, -43.89859572486944472, -4.360112732550413206 ) ) ;
#1475=CARTESIAN_POINT ( 'NONE',  ( -39.87462524744216807, -37.55140427513057944, 1.507589171976367215 ) ) ;
#1478=CARTESIAN_POINT ( 'NONE',  ( -34.53486167607238144, -30.15000000000000213, -8.900167166472096270 ) ) ;
#1484=CARTESIAN_POINT ( 'NONE',  ( -36.28032828410546529, -36.24859572486943904, 6.359104887540839357 ) ) ;
#1485=CARTESIAN_POINT ( 'NONE',  ( -22.93678734525658314, -30.75000000000000000, -7.063212654743582952 ) ) ;
#1487=CARTESIAN_POINT ( 'NONE',  ( -28.51387258211773812, -46.80000000000001137, 9.383039235653802379 ) ) ;
#1493=CARTESIAN_POINT ( 'NONE',  ( -28.72263195913613387, -42.80140427513057944, 8.403638346957361449 ) ) ;
#1498=CARTESIAN_POINT ( 'NONE',  ( -31.39812190974910422, -43.95000000000000284, 8.827394325379140483 ) ) ;
#1505=CARTESIAN_POINT ( 'NONE',  ( -21.17260567462091458, -40.05000000000001137, -1.398121909749242331 ) ) ;
#1510=CARTESIAN_POINT ( 'NONE',  ( -36.75497492228666374, -45.99859572486943904, -6.680053920257780220 ) ) ;
#1512=CARTESIAN_POINT ( 'NONE',  ( -38.46456197978948666, -35.40000000000000568, 4.312909747525784709 ) ) ;
#1516=CARTESIAN_POINT ( 'NONE',  ( -37.98859631114233792, -42.84859572486944046, -4.007875659808334490 ) ) ;
#1517=CARTESIAN_POINT ( 'NONE',  ( -31.50758917197619979, -47.94859572486943478, 9.874625247442176956 ) ) ;
#1518=CARTESIAN_POINT ( 'NONE',  ( -23.31994607974211675, -48.50140427513058938, 6.754974922286503869 ) ) ;
#1527=CARTESIAN_POINT ( 'NONE',  ( -26.18828373723858149, -31.59859572486943335, -7.597606577763319713 ) ) ;
#1528=CARTESIAN_POINT ( 'NONE',  ( -36.71751442127229836, -36.00000000000000711, -6.717514421272142044 ) ) ;
#1530=CARTESIAN_POINT ( 'NONE',  ( -25.46513832392765408, -43.64999999999999147, 8.900167166472096270 ) ) ;
#1538=CARTESIAN_POINT ( 'NONE',  ( -33.90612223281073057, -46.10140427513058370, 7.549504333439023718 ) ) ;
#1543=CARTESIAN_POINT ( 'NONE',  ( -36.31971658582311591, -44.25000000000000000, 6.319716585823200283 ) ) ;
#1547=CARTESIAN_POINT ( 'NONE',  ( -31.39812190974910422, -37.94999999999998153, 8.827394325379140483 ) ) ;
#1552=CARTESIAN_POINT ( 'NONE',  ( -36.71751442127229836, -33.00000000000000711, -6.717514421272142044 ) ) ;
#1559=CARTESIAN_POINT ( 'NONE',  ( -36.28032828410546529, -36.24859572486943904, 6.359104887540839357 ) ) ;
#1561=CARTESIAN_POINT ( 'NONE',  ( -28.49241082802385350, -46.44859572486943478, -9.874625247442173404 ) ) ;
#1562=CARTESIAN_POINT ( 'NONE',  ( -20.62524821624488069, -48.20140427513058512, 1.538452329860250378 ) ) ;
#1564=CARTESIAN_POINT ( 'NONE',  ( -25.46513832392765408, -31.65000000000000568, 8.900167166472096270 ) ) ;
#1571=CARTESIAN_POINT ( 'NONE',  ( -22.45049566656107842, -37.89859572486944472, -3.906122232810846917 ) ) ;
#1573=CARTESIAN_POINT ( 'NONE',  ( -34.31290974752564438, -44.10000000000000853, 8.464561979789547053 ) ) ;
#1577=CARTESIAN_POINT ( 'NONE',  ( -36.71751442127229836, -51.00000000000000711, -6.717514421272142044 ) ) ;
#1584=CARTESIAN_POINT ( 'NONE',  ( -38.83610826798580717, -49.55140427513056522, 1.343104241417631073 ) ) ;
#1591=( NAMED_UNIT ( * ) SI_UNIT ( $, .STERADIAN. ) SOLID_ANGLE_UNIT ( ) );
#1592=CARTESIAN_POINT ( 'NONE',  ( -34.05750781543318340, -42.15000000000001279, -7.963307464738195840 ) ) ;
#1597=CARTESIAN_POINT ( 'NONE',  ( -39.86591130483550671, -32.55000000000000426, 1.562606840307984468 ) ) ;
#1600=CARTESIAN_POINT ( 'NONE',  ( -28.51387258211773812, -43.80000000000000426, 9.383039235653802379 ) ) ;
#1605=CARTESIAN_POINT ( 'NONE',  ( -37.54950433343896776, -36.39859572486944472, 3.906122232810848249 ) ) ;
#1606=CARTESIAN_POINT ( 'NONE',  ( -25.73429323749904185, -46.59859572486944046, -8.488613101951701267 ) ) ;
#1607=CARTESIAN_POINT ( 'NONE',  ( -34.48522952044771017, -47.15140427513058086, -8.925456012876139766 ) ) ;
#1618=CARTESIAN_POINT ( 'NONE',  ( -26.18828373723858149, -40.59859572486944757, -7.597606577763319713 ) ) ;
#1619=CARTESIAN_POINT ( 'NONE',  ( -23.28248557872775137, -46.50000000000000711, 6.717514421272141156 ) ) ;
#1621=CARTESIAN_POINT ( 'NONE',  ( -20.13408869516453947, -49.04999999999999716, -1.562606840307983136 ) ) ;
#1629=CARTESIAN_POINT ( 'NONE',  ( -26.14108075221394856, -33.60000000000000142, -7.573555455601170827 ) ) ;
#1640=CARTESIAN_POINT ( 'NONE',  ( -38.82739432537914581, -41.55000000000001137, 1.398121909749243441 ) ) ;
#1644=CARTESIAN_POINT ( 'NONE',  ( -25.68709025247441602, -30.60000000000000142, -8.464561979789547053 ) ) ;
#1646=CARTESIAN_POINT ( 'NONE',  ( -34.53486167607238855, -45.15000000000000568, -8.900167166472096270 ) ) ;
#1649=DIRECTION ( 'NONE',  ( -0.7061138087190628188, 0.05297714858780522285, 0.7061138087190791390 ) ) ;
#1651=CARTESIAN_POINT ( 'NONE',  ( -23.71967171589458445, -34.74859572486943904, -6.359104887540838469 ) ) ;
#1652=CARTESIAN_POINT ( 'NONE',  ( -21.07454398712378918, -50.34859572486944046, 4.485229520447505003 ) ) ;
#1653=CARTESIAN_POINT ( 'NONE',  ( -26.09387776718931917, -32.60140427513057659, -7.549504333439021941 ) ) ;
#1664=CARTESIAN_POINT ( 'NONE',  ( -33.81171626276147890, -39.09859572486944046, 7.597606577763319713 ) ) ;
#1665=CARTESIAN_POINT ( 'NONE',  ( -38.90016716647221529, -44.85000000000001563, -4.534861676072185155 ) ) ;
#1668=CARTESIAN_POINT ( 'NONE',  ( -38.46456197978948666, -44.40000000000000568, 4.312909747525784709 ) ) ;
#1676=CARTESIAN_POINT ( 'NONE',  ( -31.32969295284206979, -30.30000000000000782, -8.395350895058669494 ) ) ;
#1684=CARTESIAN_POINT ( 'NONE',  ( -22.03669253526174998, -40.35000000000000142, 4.057507815433014642 ) ) ;
#1689=CARTESIAN_POINT ( 'NONE',  ( -38.46456197978948666, -35.40000000000000568, 4.312909747525784709 ) ) ;
#1691=CARTESIAN_POINT ( 'NONE',  ( -39.38303923565386100, -41.70000000000000995, -1.486127417882099788 ) ) ;
#1696=CARTESIAN_POINT ( 'NONE',  ( -28.65689575858256077, -37.44859572486943478, -8.836108267985801845 ) ) ;
#1697=CARTESIAN_POINT ( 'NONE',  ( -34.26570676250101855, -48.09859572486944046, 8.488613101951703044 ) ) ;
#1698=CARTESIAN_POINT ( 'NONE',  ( -25.99212434019154472, -30.65140427513057730, 7.988596311142242890 ) ) ;
#1702=CARTESIAN_POINT ( 'NONE',  ( -34.31290974752564438, -41.10000000000000142, 8.464561979789547053 ) ) ;
#1707=DIRECTION ( 'NONE',  ( 0.000000000000000000, 0.000000000000000000, 1.000000000000000000 ) ) ;
#1710=CARTESIAN_POINT ( 'NONE',  ( -33.81171626276147890, -45.09859572486944046, 7.597606577763319713 ) ) ;
#1711=CARTESIAN_POINT ( 'NONE',  ( -21.53543802021056663, -45.90000000000001279, -4.312909747525783821 ) ) ;
#1714=CARTESIAN_POINT ( 'NONE',  ( -37.10260095646111012, -31.25140427513058228, 7.023824353025939438 ) ) ;
#1722=CARTESIAN_POINT ( 'NONE',  ( -38.39535089505872634, -35.70000000000000995, -1.329692952841885267 ) ) ;
#1733=CARTESIAN_POINT ( 'NONE',  ( -36.01040764008574513, -45.00000000000000711, -6.010407640085605685 ) ) ;
#1739=CARTESIAN_POINT ( 'NONE',  ( -38.46456197978948666, -38.40000000000000568, 4.312909747525784709 ) ) ;
#1741=CARTESIAN_POINT ( 'NONE',  ( -31.56260684030781505, -40.95000000000000995, 9.865911304835508489 ) ) ;
#1746=CARTESIAN_POINT ( 'NONE',  ( -25.89286002894218086, -47.64859572486945183, 7.938018618334153231 ) ) ;
#1747=CARTESIAN_POINT ( 'NONE',  ( -20.61696076434619584, -34.20000000000000995, 1.486127417882100676 ) ) ;
#1748=CARTESIAN_POINT ( 'NONE',  ( -35.97294713907137975, -41.00140427513057517, -6.047868141099968398 ) ) ;
#1752=CARTESIAN_POINT ( 'NONE',  ( -38.90016716647221529, -32.85000000000000853, -4.534861676072185155 ) ) ;
#1758=CARTESIAN_POINT ( 'NONE',  ( -23.95213185889994989, -44.49859572486944614, 5.972947139071243861 ) ) ;
#1760=CARTESIAN_POINT ( 'NONE',  ( -20.13408869516453947, -43.04999999999999005, -1.562606840307983136 ) ) ;
#1762=CARTESIAN_POINT ( 'NONE',  ( -38.87487832006816291, -34.85140427513057659, -4.584493831696867971 ) ) ;
#1770=CARTESIAN_POINT ( 'NONE',  ( -23.68028341417693738, -36.75000000000000711, -6.319716585823198507 ) ) ;
#1772=PRODUCT_DEFINITION_CONTEXT ( 'detailed design', #8148, 'design' ) ;
#1783=CARTESIAN_POINT ( 'NONE',  ( -34.53486167607238855, -39.14999999999999858, -8.900167166472096270 ) ) ;
#1785=CARTESIAN_POINT ( 'NONE',  ( -36.75497492228666374, -30.99859572486944259, -6.680053920257780220 ) ) ;
#1786=CARTESIAN_POINT ( 'NONE',  ( -39.86591130483550671, -32.55000000000000426, 1.562606840307984468 ) ) ;
#1787=CARTESIAN_POINT ( 'NONE',  ( -28.72263195913613387, -42.80140427513057944, 8.403638346957361449 ) ) ;
#1791=CARTESIAN_POINT ( 'NONE',  ( -28.43739315969223824, -36.45000000000000284, -9.865911304835512041 ) ) ;
#1798=CARTESIAN_POINT ( 'NONE',  ( -28.49241082802385350, -34.44859572486944188, -9.874625247442173404 ) ) ;
#1799=CARTESIAN_POINT ( 'NONE',  ( -39.38303923565386100, -50.70000000000000995, -1.486127417882099788 ) ) ;
#1803=CARTESIAN_POINT ( 'NONE',  ( -20.62524821624488069, -36.20140427513057091, 1.538452329860250378 ) ) ;
#1810=CARTESIAN_POINT ( 'NONE',  ( -33.85891924778610473, -41.10000000000000142, 7.573555455601171715 ) ) ;
#1823=CARTESIAN_POINT ( 'NONE',  ( -20.13408869516454303, -49.05000000000000426, -1.562606840307982692 ) ) ;
#1826=CARTESIAN_POINT ( 'NONE',  ( -31.34310424141748896, -47.94859572486943478, 8.836108267985801845 ) ) ;
#1827=CARTESIAN_POINT ( 'NONE',  ( -38.90016716647221529, -32.85000000000000853, -4.534861676072185155 ) ) ;
#1828=CARTESIAN_POINT ( 'NONE',  ( -26.09387776718931917, -41.60140427513058370, -7.549504333439021941 ) ) ;
#1831=CARTESIAN_POINT ( 'NONE',  ( -34.58449383169706692, -34.14859572486943051, -8.874878320068054549 ) ) ;
#1832=CARTESIAN_POINT ( 'NONE',  ( -28.43739315969223824, -39.45000000000000995, -9.865911304835512041 ) ) ;
#1841=CARTESIAN_POINT ( 'NONE',  ( -36.75497492228666374, -30.99859572486944259, -6.680053920257780220 ) ) ;
#1842=CARTESIAN_POINT ( 'NONE',  ( -37.06321265474346660, -50.24999999999998579, 7.063212654743582952 ) ) ;
#1846=CARTESIAN_POINT ( 'NONE',  ( -34.48522952044771017, -38.15140427513058086, -8.925456012876139766 ) ) ;
#1853=CARTESIAN_POINT ( 'NONE',  ( -33.85891924778610473, -44.10000000000000853, 7.573555455601171715 ) ) ;
#1859=CARTESIAN_POINT ( 'NONE',  ( -25.99212434019154472, -36.65140427513058086, 7.988596311142242890 ) ) ;
#1863=CARTESIAN_POINT ( 'NONE',  ( -22.03669253526174998, -34.35000000000000853, 4.057507815433014642 ) ) ;
#1865=CARTESIAN_POINT ( 'NONE',  ( -20.13408869516454303, -46.05000000000000426, -1.562606840307982692 ) ) ;
#1868=CARTESIAN_POINT ( 'NONE',  ( -21.18131961722757595, -50.04859572486944330, -1.453139578080854699 ) ) ;
#1869=CARTESIAN_POINT ( 'NONE',  ( -31.56260684030781505, -34.95000000000000995, 9.865911304835510265 ) ) ;
#1871=CARTESIAN_POINT ( 'NONE',  ( -28.54686042191934092, -41.45140427513058512, -8.818680382772479120 ) ) ;
#1874=CARTESIAN_POINT ( 'NONE',  ( -38.44051085762733777, -39.39859572486943762, 4.360112732550414982 ) ) ;
#1875=CARTESIAN_POINT ( 'NONE',  ( -38.46456197978948666, -32.40000000000000568, 4.312909747525784709 ) ) ;
#1882=CARTESIAN_POINT ( 'NONE',  ( -38.81868038277247734, -51.54859572486944330, 1.453139578080855365 ) ) ;
#1883=CARTESIAN_POINT ( 'NONE',  ( -34.36011273255026310, -34.10140427513057659, 8.440510857627391061 ) ) ;
#1888=CARTESIAN_POINT ( 'NONE',  ( -20.62524821624488069, -39.20140427513058512, 1.538452329860250378 ) ) ;
#1895=CARTESIAN_POINT ( 'NONE',  ( -36.01040764008574513, -42.00000000000000711, -6.010407640085605685 ) ) ;
#1899=CARTESIAN_POINT ( 'NONE',  ( -36.71751442127229836, -48.00000000000000711, -6.717514421272142044 ) ) ;
#1902=CARTESIAN_POINT ( 'NONE',  ( -23.64089511245930098, -29.75140427513057517, -6.280328284105564762 ) ) ;
#1904=CARTESIAN_POINT ( 'NONE',  ( -28.60187809025093841, -33.45000000000000995, -8.827394325379140483 ) ) ;
#1909=CARTESIAN_POINT ( 'NONE',  ( -28.51387258211773812, -40.80000000000000426, 9.383039235653802379 ) ) ;
#1910=CARTESIAN_POINT ( 'NONE',  ( -34.00787565980851213, -44.15140427513058086, -7.988596311142238449 ) ) ;
#1914=CARTESIAN_POINT ( 'NONE',  ( -31.50758917197619979, -38.94859572486943478, 9.874625247442176956 ) ) ;
#1915=CARTESIAN_POINT ( 'NONE',  ( -34.53486167607238144, -42.15000000000001279, -8.900167166472096270 ) ) ;
#1921=CARTESIAN_POINT ( 'NONE',  ( -21.07454398712378918, -32.34859572486942625, 4.485229520447505003 ) ) ;
#1922=CARTESIAN_POINT ( 'NONE',  ( -20.61696076434619584, -49.20000000000000995, 1.486127417882100676 ) ) ;
#1928=CARTESIAN_POINT ( 'NONE',  ( -37.10260095646111012, -49.25140427513058938, 7.023824353025939438 ) ) ;
#1936=CARTESIAN_POINT ( 'NONE',  ( -37.57355545560112375, -41.40000000000000568, 3.858919247786223305 ) ) ;
#1941=CARTESIAN_POINT ( 'NONE',  ( -21.53543802021056663, -45.90000000000001279, -4.312909747525783821 ) ) ;
#1944=CARTESIAN_POINT ( 'NONE',  ( -26.09387776718931917, -32.60140427513057659, -7.549504333439021941 ) ) ;
#1946=CARTESIAN_POINT ( 'NONE',  ( -37.96330746473829976, -35.85000000000000142, -4.057507815433013754 ) ) ;
#1952=CARTESIAN_POINT ( 'NONE',  ( -38.90016716647221529, -41.84999999999999432, -4.534861676072185155 ) ) ;
#1953=CARTESIAN_POINT ( 'NONE',  ( -37.93801861833426159, -49.85140427513058370, -4.107139971057695682 ) ) ;
#1956=CARTESIAN_POINT ( 'NONE',  ( -28.46154767013959486, -32.79859572486943620, 9.374751783755112200 ) ) ;
#1962=CARTESIAN_POINT ( 'NONE',  ( -22.03669253526174998, -46.34999999999998721, 4.057507815433014642 ) ) ;
#1963=CARTESIAN_POINT ( 'NONE',  ( -26.18828373723858149, -49.59859572486944046, -7.597606577763319713 ) ) ;
#1964=CARTESIAN_POINT ( 'NONE',  ( -34.31290974752564438, -50.10000000000000853, 8.464561979789547053 ) ) ;
#1967=CARTESIAN_POINT ( 'NONE',  ( -23.31994607974211675, -42.50140427513057517, 6.754974922286503869 ) ) ;
#1968=DIRECTION ( 'NONE',  ( 0.7061138087190598212, -0.05297714858780431385, -0.7061138087190823587 ) ) ;
#1976=CARTESIAN_POINT ( 'NONE',  ( -21.60464910494133406, -46.20000000000000284, 1.329692952841886155 ) ) ;
#1983=CARTESIAN_POINT ( 'NONE',  ( -20.13408869516453947, -46.05000000000001137, -1.562606840307983136 ) ) ;
#1986=CARTESIAN_POINT ( 'NONE',  ( -38.83610826798580717, -31.55140427513057588, 1.343104241417631073 ) ) ;
#1990=CARTESIAN_POINT ( 'NONE',  ( -31.39812190974910422, -34.95000000000000995, 8.827394325379140483 ) ) ;
#1992=CARTESIAN_POINT ( 'NONE',  ( -25.46513832392766119, -49.64999999999999858, 8.900167166472096270 ) ) ;
#1996=CARTESIAN_POINT ( 'NONE',  ( -23.28248557872775137, -43.50000000000001421, 6.717514421272141156 ) ) ;
#1997=CARTESIAN_POINT ( 'NONE',  ( -25.94249218456686279, -31.65000000000000568, 7.963307464738195840 ) ) ;
#2001=CARTESIAN_POINT ( 'NONE',  ( -34.26570676250101855, -33.09859572486943335, 8.488613101951703044 ) ) ;
#2009=CARTESIAN_POINT ( 'NONE',  ( -31.32969295284206979, -45.30000000000000426, -8.395350895058669494 ) ) ;
#2010=CARTESIAN_POINT ( 'NONE',  ( -34.58449383169706692, -40.14859572486943762, -8.874878320068054549 ) ) ;
#2011=CARTESIAN_POINT ( 'NONE',  ( -31.61762450863942320, -39.95140427513058512, 9.857197362228843573 ) ) ;
#2015=CARTESIAN_POINT ( 'NONE',  ( -39.87462524744216807, -43.55140427513057944, 1.507589171976367215 ) ) ;
#2023=CARTESIAN_POINT ( 'NONE',  ( -38.81868038277247734, -33.54859572486944330, 1.453139578080855365 ) ) ;
#2024=CARTESIAN_POINT ( 'NONE',  ( -23.28248557872775137, -31.50000000000000711, 6.717514421272141156 ) ) ;
#2030=CARTESIAN_POINT ( 'NONE',  ( -25.68709025247441602, -39.60000000000000853, -8.464561979789547053 ) ) ;
#2033=CARTESIAN_POINT ( 'NONE',  ( -31.27736804086391942, -32.30140427513056522, -8.403638346957361449 ) ) ;
#2036=CARTESIAN_POINT ( 'NONE',  ( -22.03669253526174998, -49.35000000000000853, 4.057507815433014642 ) ) ;
#2042=CARTESIAN_POINT ( 'NONE',  ( -39.38303923565386100, -44.70000000000000284, -1.486127417882099788 ) ) ;
#2043=CARTESIAN_POINT ( 'NONE',  ( -36.35910488754074521, -46.25140427513058228, 6.280328284105565650 ) ) ;
#2047=CARTESIAN_POINT ( 'NONE',  ( -23.24502507771338600, -47.49859572486944614, 6.680053920257780220 ) ) ;
#2049=CARTESIAN_POINT ( 'NONE',  ( -25.46513832392766119, -31.65000000000000568, 8.900167166472096270 ) ) ;
#2055=CARTESIAN_POINT ( 'NONE',  ( -34.05750781543318340, -48.15000000000001279, -7.963307464738195840 ) ) ;
#2056=CARTESIAN_POINT ( 'NONE',  ( -36.75497492228666374, -36.99859572486943193, -6.680053920257780220 ) ) ;
#2057=CARTESIAN_POINT ( 'NONE',  ( -20.62524821624488069, -45.20140427513059223, 1.538452329860250378 ) ) ;
#2060=CARTESIAN_POINT ( 'NONE',  ( -25.63988726744978663, -41.60140427513058370, -8.440510857627391061 ) ) ;
#2069=CARTESIAN_POINT ( 'NONE',  ( -22.01140368885771892, -35.34859572486944046, 4.007875659808335378 ) ) ;
#2070=CARTESIAN_POINT ( 'NONE',  ( -28.51387258211773812, -31.80000000000000782, 9.383039235653802379 ) ) ;
#2075=CARTESIAN_POINT ( 'NONE',  ( -38.46456197978948666, -41.40000000000000568, 4.312909747525784709 ) ) ;
#2078=CARTESIAN_POINT ( 'NONE',  ( -21.61293655684001536, -48.20140427513058512, 1.382017864820032971 ) ) ;
#2083=CARTESIAN_POINT ( 'NONE',  ( -26.14108075221394856, -42.60000000000000853, -7.573555455601170827 ) ) ;
#2091=CARTESIAN_POINT ( 'NONE',  ( -37.06321265474346660, -47.25000000000000711, 7.063212654743582952 ) ) ;
#2092=CARTESIAN_POINT ( 'NONE',  ( -38.39535089505872634, -32.70000000000000995, -1.329692952841885267 ) ) ;
#2096=CARTESIAN_POINT ( 'NONE',  ( -20.60867331244750034, -47.19859572486943478, 1.433802505903951419 ) ) ;
#2098=CARTESIAN_POINT ( 'NONE',  ( -20.13408869516454303, -31.05000000000000426, -1.562606840307982692 ) ) ;
#2102=CARTESIAN_POINT ( 'NONE',  ( -22.42644454439892598, -48.90000000000000568, -3.858919247786222861 ) ) ;
#2104=CARTESIAN_POINT ( 'NONE',  ( -31.53845232986046554, -37.29859572486943620, -9.374751783755117529 ) ) ;
#2105=CARTESIAN_POINT ( 'NONE',  ( -37.10260095646111012, -40.25140427513058228, 7.023824353025939438 ) ) ;
#2106=CLOSED_SHELL ( 'NONE', ( #6255, #4257, #3642, #3016 ) ) ;
#2109=CARTESIAN_POINT ( 'NONE',  ( -39.37475178375516549, -43.70140427513058512, -1.538452329860249712 ) ) ;
#2116=CARTESIAN_POINT ( 'NONE',  ( -37.54950433343896776, -33.39859572486943762, 3.906122232810848249 ) ) ;
#2117=CARTESIAN_POINT ( 'NONE',  ( -22.93678734525658314, -36.75000000000000711, -7.063212654743582952 ) ) ;
#2123=CARTESIAN_POINT ( 'NONE',  ( -38.46456197978948666, -50.40000000000000568, 4.312909747525784709 ) ) ;
#2128=CARTESIAN_POINT ( 'NONE',  ( -24.02705286092866643, -39.50140427513058228, 6.047868141099968398 ) ) ;
#2131=CARTESIAN_POINT ( 'NONE',  ( -28.60187809025093841, -42.45000000000000284, -8.827394325379140483 ) ) ;
#2137=CARTESIAN_POINT ( 'NONE',  ( -38.46456197978948666, -50.40000000000000568, 4.312909747525784709 ) ) ;
#2138=CARTESIAN_POINT ( 'NONE',  ( -28.60187809025093841, -33.45000000000000995, -8.827394325379140483 ) ) ;
#2142=CARTESIAN_POINT ( 'NONE',  ( -34.58449383169706692, -49.14859572486945183, -8.874878320068054549 ) ) ;
#2147=CARTESIAN_POINT ( 'NONE',  ( -23.68028341417693738, -48.75000000000001421, -6.319716585823198507 ) ) ;
#2148=CARTESIAN_POINT ( 'NONE',  ( -28.46154767013959486, -38.79859572486943620, 9.374751783755112200 ) ) ;
#2149=CARTESIAN_POINT ( 'NONE',  ( -39.87462524744216807, -43.55140427513057944, 1.507589171976367215 ) ) ;
#2160=CARTESIAN_POINT ( 'NONE',  ( -28.61798213517984024, -35.79859572486943620, 8.387063443159973986 ) ) ;
#2161=CARTESIAN_POINT ( 'NONE',  ( -31.56260684030781505, -34.95000000000000995, 9.865911304835510265 ) ) ;
#2165=CARTESIAN_POINT ( 'NONE',  ( -38.46456197978948666, -47.40000000000001279, 4.312909747525784709 ) ) ;
#2170=CARTESIAN_POINT ( 'NONE',  ( -23.64089511245930098, -41.75140427513057517, -6.280328284105564762 ) ) ;
#2173=CARTESIAN_POINT ( 'NONE',  ( -25.94249218456686279, -40.65000000000000568, 7.963307464738194952 ) ) ;
#2180=CARTESIAN_POINT ( 'NONE',  ( -36.31971658582311591, -38.25000000000001421, 6.319716585823199395 ) ) ;
#2183=CARTESIAN_POINT ( 'NONE',  ( -38.44051085762733777, -51.39859572486944472, 4.360112732550414982 ) ) ;
#2185=CARTESIAN_POINT ( 'NONE',  ( -28.43739315969223824, -30.44999999999999574, -9.865911304835512041 ) ) ;
#2190=CARTESIAN_POINT ( 'NONE',  ( -23.71967171589458445, -40.74859572486943904, -6.359104887540838469 ) ) ;
#2191=CARTESIAN_POINT ( 'NONE',  ( -34.58449383169706692, -37.14859572486943762, -8.874878320068054549 ) ) ;
#2192=CARTESIAN_POINT ( 'NONE',  ( -35.97294713907137975, -32.00140427513057517, -6.047868141099968398 ) ) ;
#2204=CARTESIAN_POINT ( 'NONE',  ( -26.14108075221394856, -48.60000000000000142, -7.573555455601170827 ) ) ;
#2205=CARTESIAN_POINT ( 'NONE',  ( -25.46513832392765408, -34.64999999999998437, 8.900167166472096270 ) ) ;
#2207=CARTESIAN_POINT ( 'NONE',  ( -20.61696076434619584, -49.20000000000000995, 1.486127417882100676 ) ) ;
#2214=CARTESIAN_POINT ( 'NONE',  ( -36.35910488754074521, -40.25140427513058228, 6.280328284105565650 ) ) ;
#2220=CARTESIAN_POINT ( 'NONE',  ( -21.17260567462091103, -43.04999999999999716, -1.398121909749241887 ) ) ;
#2225=CARTESIAN_POINT ( 'NONE',  ( -22.42644454439892598, -42.90000000000000568, -3.858919247786222861 ) ) ;
#2230=CARTESIAN_POINT ( 'NONE',  ( -38.90016716647221529, -32.85000000000000853, -4.534861676072185155 ) ) ;
#2231=DIRECTION ( 'NONE',  ( -0.7071067811865587860, 0.000000000000000000, -0.7071067811865362485 ) ) ;
#2232=CARTESIAN_POINT ( 'NONE',  ( -39.38303923565386100, -35.70000000000000995, -1.486127417882099788 ) ) ;
#2236=CARTESIAN_POINT ( 'NONE',  ( -21.18131961722757595, -44.04859572486944330, -1.453139578080854699 ) ) ;
#2238=CARTESIAN_POINT ( 'NONE',  ( -28.46154767013959486, -47.79859572486944330, 9.374751783755112200 ) ) ;
#2239=CARTESIAN_POINT ( 'NONE',  ( -25.99212434019154472, -33.65140427513057375, 7.988596311142242890 ) ) ;
#2242=CARTESIAN_POINT ( 'NONE',  ( -25.68709025247441602, -30.60000000000000142, -8.464561979789547053 ) ) ;
#2248=CARTESIAN_POINT ( 'NONE',  ( -23.95213185889994989, -41.49859572486943904, 5.972947139071243861 ) ) ;
#2249=CARTESIAN_POINT ( 'NONE',  ( -20.13408869516453947, -40.05000000000001137, -1.562606840307983136 ) ) ;
#2251=CARTESIAN_POINT ( 'NONE',  ( -39.86591130483550671, -50.55000000000001137, 1.562606840307984468 ) ) ;
#2259=CARTESIAN_POINT ( 'NONE',  ( -21.16389173201424612, -48.05140427513057233, -1.343104241417630185 ) ) ;
#2267=PRESENTATION_STYLE_ASSIGNMENT (( #3502 ) ) ;
#2269=CARTESIAN_POINT ( 'NONE',  ( -23.68028341417693738, -33.75000000000001421, -6.319716585823198507 ) ) ;
#2272=CARTESIAN_POINT ( 'NONE',  ( -28.43739315969223824, -33.45000000000000995, -9.865911304835512041 ) ) ;
#2275=CARTESIAN_POINT ( 'NONE',  ( -20.13408869516454303, -40.05000000000001137, -1.562606840307982692 ) ) ;
#2279=CARTESIAN_POINT ( 'NONE',  ( -21.18131961722757595, -35.04859572486943620, -1.453139578080854699 ) ) ;
#2280=CARTESIAN_POINT ( 'NONE',  ( -38.44051085762733777, -48.39859572486944472, 4.360112732550414982 ) ) ;
#2281=CARTESIAN_POINT ( 'NONE',  ( -36.35910488754074521, -31.25140427513058228, 6.280328284105565650 ) ) ;
#2291=CARTESIAN_POINT ( 'NONE',  ( -28.65689575858256077, -43.44859572486944188, -8.836108267985801845 ) ) ;
#2292=CARTESIAN_POINT ( 'NONE',  ( -23.28248557872775137, -40.50000000000000711, 6.717514421272141156 ) ) ;
#2296=CARTESIAN_POINT ( 'NONE',  ( -22.89739904353894318, -29.75140427513057517, -7.023824353025938549 ) ) ;
#2303=CARTESIAN_POINT ( 'NONE',  ( -36.35910488754074521, -49.25140427513058938, 6.280328284105565650 ) ) ;
#2314=CARTESIAN_POINT ( 'NONE',  ( -38.82739432537914581, -38.54999999999999716, 1.398121909749243441 ) ) ;
#2317=CARTESIAN_POINT ( 'NONE',  ( -21.53543802021056663, -33.90000000000000568, -4.312909747525783821 ) ) ;
#2320=CARTESIAN_POINT ( 'NONE',  ( -39.86591130483550671, -44.55000000000000426, 1.562606840307984690 ) ) ;
#2324=CARTESIAN_POINT ( 'NONE',  ( -36.28032828410546529, -42.24859572486943904, 6.359104887540839357 ) ) ;
#2325=CARTESIAN_POINT ( 'NONE',  ( -38.92545601287626056, -48.84859572486942625, -4.485229520447501450 ) ) ;
#2326=CARTESIAN_POINT ( 'NONE',  ( -34.00787565980851213, -32.15140427513058086, -7.988596311142238449 ) ) ;
#2330=CARTESIAN_POINT ( 'NONE',  ( -34.31290974752564438, -32.10000000000000142, 8.464561979789547053 ) ) ;
#2335=CARTESIAN_POINT ( 'NONE',  ( -25.89286002894218086, -41.64859572486943762, 7.938018618334153231 ) ) ;
#2336=CARTESIAN_POINT ( 'NONE',  ( -36.71751442127229836, -45.00000000000000711, -6.717514421272142044 ) ) ;
#2338=CARTESIAN_POINT ( 'NONE',  ( -25.51477047955235378, -30.65140427513057730, 8.925456012876139766 ) ) ;
#2346=CARTESIAN_POINT ( 'NONE',  ( -21.60464910494133406, -31.20000000000000639, 1.329692952841886155 ) ) ;
#2356=CARTESIAN_POINT ( 'NONE',  ( -31.32969295284206979, -36.30000000000000426, -8.395350895058669494 ) ) ;
#2360=CARTESIAN_POINT ( 'NONE',  ( -21.53543802021056663, -30.90000000000000924, -4.312909747525783821 ) ) ;
#2363=CARTESIAN_POINT ( 'NONE',  ( -25.46513832392766119, -37.65000000000000568, 8.900167166472096270 ) ) ;
#2365=SHAPE_REPRESENTATION_RELATIONSHIP ( 'NONE' , 'NONE' ,  #7373, #7808 ) ;
#2368=CARTESIAN_POINT ( 'NONE',  ( -25.89286002894218086, -35.64859572486943051, 7.938018618334153231 ) ) ;
#2369=CARTESIAN_POINT ( 'NONE',  ( -28.46154767013959486, -44.79859572486943620, 9.374751783755112200 ) ) ;
#2370=CARTESIAN_POINT ( 'NONE',  ( -31.45313957808072303, -33.95140427513058512, 8.818680382772479120 ) ) ;
#2375=CARTESIAN_POINT ( 'NONE',  ( -23.28248557872775137, -40.50000000000000711, 6.717514421272141156 ) ) ;
#2381=CARTESIAN_POINT ( 'NONE',  ( -25.89286002894218086, -44.64859572486944472, 7.938018618334153231 ) ) ;
#2382=CARTESIAN_POINT ( 'NONE',  ( -39.86591130483550671, -47.54999999999999716, 1.562606840307984468 ) ) ;
#2385=CARTESIAN_POINT ( 'NONE',  ( -28.56619749409589204, -36.80140427513057944, 9.391326687552490782 ) ) ;
#2392=CARTESIAN_POINT ( 'NONE',  ( -26.14108075221394856, -36.60000000000000853, -7.573555455601170827 ) ) ;
#2398=CARTESIAN_POINT ( 'NONE',  ( -38.82739432537914581, -44.55000000000001137, 1.398121909749243441 ) ) ;
#2403=CARTESIAN_POINT ( 'NONE',  ( -34.53486167607238144, -36.15000000000001279, -8.900167166472096270 ) ) ;
#2405=CARTESIAN_POINT ( 'NONE',  ( -39.86591130483550671, -38.55000000000000426, 1.562606840307984690 ) ) ;
#2407=CARTESIAN_POINT ( 'NONE',  ( -37.98859631114233792, -48.84859572486942625, -4.007875659808334490 ) ) ;
#2408=CARTESIAN_POINT ( 'NONE',  ( -36.71751442127229836, -30.00000000000000711, -6.717514421272142044 ) ) ;
#2409=CARTESIAN_POINT ( 'NONE',  ( -31.45313957808072303, -36.95140427513057801, 8.818680382772479120 ) ) ;
#2414=CARTESIAN_POINT ( 'NONE',  ( -39.38303923565386100, -41.70000000000000995, -1.486127417882099788 ) ) ;
#2420=CARTESIAN_POINT ( 'NONE',  ( -36.28032828410546529, -39.24859572486943904, 6.359104887540839357 ) ) ;
#2421=CARTESIAN_POINT ( 'NONE',  ( -21.53543802021056663, -48.90000000000000568, -4.312909747525783821 ) ) ;
#2423=CARTESIAN_POINT ( 'NONE',  ( -22.89739904353894318, -35.75140427513057517, -7.023824353025938549 ) ) ;
#2431=CARTESIAN_POINT ( 'NONE',  ( -21.17260567462091458, -34.04999999999998295, -1.398121909749242331 ) ) ;
#2445=CARTESIAN_POINT ( 'NONE',  ( -38.90016716647221529, -38.85000000000000853, -4.534861676072185155 ) ) ;
#2448=CARTESIAN_POINT ( 'NONE',  ( -22.45049566656107842, -46.89859572486944472, -3.906122232810846917 ) ) ;
#2449=CARTESIAN_POINT ( 'NONE',  ( -25.68709025247441602, -33.60000000000000142, -8.464561979789547053 ) ) ;
#2450=CARTESIAN_POINT ( 'NONE',  ( -38.83610826798580717, -37.55140427513057944, 1.343104241417631073 ) ) ;
#2453=CARTESIAN_POINT ( 'NONE',  ( -21.09983283352784156, -37.35000000000000853, 4.534861676072186043 ) ) ;
#2459=CARTESIAN_POINT ( 'NONE',  ( -38.92545601287626056, -33.84859572486942625, -4.485229520447501450 ) ) ;
#2460=CARTESIAN_POINT ( 'NONE',  ( -31.61762450863942320, -30.95140427513058157, 9.857197362228843573 ) ) ;
#2463=CARTESIAN_POINT ( 'NONE',  ( -39.37475178375516549, -37.70140427513057091, -1.538452329860249712 ) ) ;
#2471=CARTESIAN_POINT ( 'NONE',  ( -33.85891924778610473, -38.10000000000000853, 7.573555455601171715 ) ) ;
#2485=CARTESIAN_POINT ( 'NONE',  ( -31.56260684030781505, -49.95000000000000995, 9.865911304835508489 ) ) ;
#2487=CARTESIAN_POINT ( 'NONE',  ( -23.24502507771338600, -32.49859572486943904, 6.680053920257780220 ) ) ;
#2488=CARTESIAN_POINT ( 'NONE',  ( -25.46513832392765408, -34.64999999999998437, 8.900167166472096270 ) ) ;
#2489=CARTESIAN_POINT ( 'NONE',  ( -34.00787565980851213, -41.15140427513058086, -7.988596311142238449 ) ) ;
#2493=CARTESIAN_POINT ( 'NONE',  ( -37.02382435302582309, -39.24859572486943904, 7.102600956461226467 ) ) ;
#2494=CARTESIAN_POINT ( 'NONE',  ( -31.56260684030781505, -37.94999999999998153, 9.865911304835510265 ) ) ;
#2503=CARTESIAN_POINT ( 'NONE',  ( -25.89286002894218086, -47.64859572486945183, 7.938018618334153231 ) ) ;
#2504=CARTESIAN_POINT ( 'NONE',  ( -36.68005392025794009, -35.00140427513057517, -6.754974922286504757 ) ) ;
#2508=CARTESIAN_POINT ( 'NONE',  ( -37.10260095646111012, -37.25140427513058228, 7.023824353025939438 ) ) ;
#2516=CARTESIAN_POINT ( 'NONE',  ( -31.32969295284206979, -45.30000000000000426, -8.395350895058669494 ) ) ;
#2520=CARTESIAN_POINT ( 'NONE',  ( -26.09387776718931917, -29.60140427513057659, -7.549504333439021941 ) ) ;
#2523=CARTESIAN_POINT ( 'NONE',  ( -23.98959235991431171, -31.50000000000000711, 6.010407640085604797 ) ) ;
#2525=CARTESIAN_POINT ( 'NONE',  ( -34.53486167607238855, -48.15000000000001279, -8.900167166472096270 ) ) ;
#2529=CARTESIAN_POINT ( 'NONE',  ( -38.40363834695740053, -48.69859572486944188, -1.277368040863739118 ) ) ;
#2530=CARTESIAN_POINT ( 'NONE',  ( -31.48612741788231517, -33.30000000000000426, -9.383039235653804155 ) ) ;
#2531=CARTESIAN_POINT ( 'NONE',  ( -36.35910488754074521, -37.25140427513058228, 6.280328284105565650 ) ) ;
#2534=CARTESIAN_POINT ( 'NONE',  ( -23.24502507771338600, -41.49859572486943904, 6.680053920257780220 ) ) ;
#2535=CARTESIAN_POINT ( 'NONE',  ( -31.48612741788231517, -39.30000000000001137, -9.383039235653804155 ) ) ;
#2543=CARTESIAN_POINT ( 'NONE',  ( -25.73429323749904185, -34.59859572486944046, -8.488613101951701267 ) ) ;
#2544=CARTESIAN_POINT ( 'NONE',  ( -36.68005392025794009, -32.00140427513057517, -6.754974922286504757 ) ) ;
#2547=CARTESIAN_POINT ( 'NONE',  ( -39.87462524744216807, -31.55140427513057588, 1.507589171976367215 ) ) ;
#2554=AXIS2_PLACEMENT_3D ( 'NONE', #7787, #1707, #3692 ) ;
#2555=CARTESIAN_POINT ( 'NONE',  ( -34.05750781543318340, -45.14999999999999858, -7.963307464738195840 ) ) ;
#2560=CARTESIAN_POINT ( 'NONE',  ( -36.71751442127229836, -42.00000000000000711, -6.717514421272142044 ) ) ;
#2563=CARTESIAN_POINT ( 'NONE',  ( -22.40239342223677355, -32.90140427513058086, -3.811716262761597473 ) ) ;
#2570=CARTESIAN_POINT ( 'NONE',  ( -33.85891924778610473, -32.10000000000000142, 7.573555455601171715 ) ) ;
#2577=CARTESIAN_POINT ( 'NONE',  ( -37.54950433343896776, -51.39859572486944472, 3.906122232810848249 ) ) ;
#2578=CARTESIAN_POINT ( 'NONE',  ( -38.46456197978948666, -32.40000000000000568, 4.312909747525784709 ) ) ;
#2580=CARTESIAN_POINT ( 'NONE',  ( -37.93801861833426159, -40.85140427513057659, -4.107139971057695682 ) ) ;
#2583=CARTESIAN_POINT ( 'NONE',  ( -36.75497492228666374, -36.99859572486943193, -6.680053920257780220 ) ) ;
#2584=CARTESIAN_POINT ( 'NONE',  ( -21.09983283352784156, -43.35000000000000853, 4.534861676072186043 ) ) ;
#2591=CARTESIAN_POINT ( 'NONE',  ( -31.53845232986046554, -31.29859572486943975, -9.374751783755117529 ) ) ;
#2592=CARTESIAN_POINT ( 'NONE',  ( -22.89739904353894318, -35.75140427513057517, -7.023824353025938549 ) ) ;
#2595=CARTESIAN_POINT ( 'NONE',  ( -20.12537475255788522, -48.05140427513057233, -1.507589171976365439 ) ) ;
#2603=CARTESIAN_POINT ( 'NONE',  ( -37.96330746473829976, -41.84999999999999432, -4.057507815433013754 ) ) ;
#2607=CARTESIAN_POINT ( 'NONE',  ( -23.28248557872775137, -40.50000000000000711, 6.717514421272141156 ) ) ;
#2610=CARTESIAN_POINT ( 'NONE',  ( -24.02705286092866643, -30.50140427513058583, 6.047868141099968398 ) ) ;
#2613=CARTESIAN_POINT ( 'NONE',  ( -23.98959235991431171, -40.50000000000000711, 6.010407640085604797 ) ) ;
#2615=CARTESIAN_POINT ( 'NONE',  ( -25.46513832392766119, -46.65000000000001279, 8.900167166472096270 ) ) ;
#2619=CARTESIAN_POINT ( 'NONE',  ( -28.43739315969223824, -42.44999999999999574, -9.865911304835512041 ) ) ;
#2620=CARTESIAN_POINT ( 'NONE',  ( -21.60464910494133406, -31.20000000000000639, 1.329692952841886155 ) ) ;
#2624=CARTESIAN_POINT ( 'NONE',  ( -39.39132668755255651, -39.69859572486944188, -1.433802505903950308 ) ) ;
#2631=CARTESIAN_POINT ( 'NONE',  ( -25.89286002894218086, -32.64859572486943762, 7.938018618334153231 ) ) ;
#2632=CARTESIAN_POINT ( 'NONE',  ( -28.61798213517984024, -50.79859572486945041, 8.387063443159973986 ) ) ;
#2633=CARTESIAN_POINT ( 'NONE',  ( -23.31994607974211675, -36.50140427513057517, 6.754974922286503869 ) ) ;
#2637=CARTESIAN_POINT ( 'NONE',  ( -21.12512167993187973, -45.35140427513057659, 4.584493831696868860 ) ) ;
#2647=CARTESIAN_POINT ( 'NONE',  ( -36.01040764008574513, -39.00000000000000711, -6.010407640085605685 ) ) ;
#2653=CARTESIAN_POINT ( 'NONE',  ( -25.68709025247441602, -48.60000000000000142, -8.464561979789547053 ) ) ;
#2656=CARTESIAN_POINT ( 'NONE',  ( -31.27736804086391942, -29.30140427513058299, -8.403638346957361449 ) ) ;
#2659=CARTESIAN_POINT ( 'NONE',  ( -37.57355545560112375, -35.40000000000000568, 3.858919247786223305 ) ) ;
#2665=CARTESIAN_POINT ( 'NONE',  ( -34.53486167607238144, -42.15000000000001279, -8.900167166472096270 ) ) ;
#2666=CARTESIAN_POINT ( 'NONE',  ( -33.90612223281073057, -49.10140427513058370, 7.549504333439023718 ) ) ;
#2669=CARTESIAN_POINT ( 'NONE',  ( -28.46154767013959486, -38.79859572486943620, 9.374751783755112200 ) ) ;
#2675=CARTESIAN_POINT ( 'NONE',  ( -33.81171626276147890, -33.09859572486943335, 7.597606577763319713 ) ) ;
#2676=CARTESIAN_POINT ( 'NONE',  ( -22.97617564697422665, -40.74859572486943904, -7.102600956461224690 ) ) ;
#2677=CARTESIAN_POINT ( 'NONE',  ( -34.48522952044771017, -41.15140427513058086, -8.925456012876139766 ) ) ;
#2681=CARTESIAN_POINT ( 'NONE',  ( -23.31994607974211675, -48.50140427513058938, 6.754974922286503869 ) ) ;
#2689=CARTESIAN_POINT ( 'NONE',  ( -25.89286002894218086, -32.64859572486943762, 7.938018618334153231 ) ) ;
#2690=CARTESIAN_POINT ( 'NONE',  ( -21.09983283352784156, -31.34999999999999787, 4.534861676072186043 ) ) ;
#2696=CARTESIAN_POINT ( 'NONE',  ( -39.38303923565386100, -41.70000000000000995, -1.486127417882099788 ) ) ;
#2698=CARTESIAN_POINT ( 'NONE',  ( -38.83610826798580717, -34.55140427513057233, 1.343104241417631073 ) ) ;
#2701=CARTESIAN_POINT ( 'NONE',  ( -38.82739432537914581, -35.55000000000000426, 1.398121909749243663 ) ) ;
#2707=CARTESIAN_POINT ( 'NONE',  ( -36.71751442127229836, -42.00000000000000711, -6.717514421272142044 ) ) ;
#2708=CARTESIAN_POINT ( 'NONE',  ( -26.14108075221394856, -30.60000000000000142, -7.573555455601170827 ) ) ;
#2711=CARTESIAN_POINT ( 'NONE',  ( -36.75497492228666374, -48.99859572486944614, -6.680053920257780220 ) ) ;
#2718=CARTESIAN_POINT ( 'NONE',  ( -23.98959235991431171, -46.50000000000000711, 6.010407640085604797 ) ) ;
#2719=CARTESIAN_POINT ( 'NONE',  ( -39.39132668755255651, -42.69859572486944188, -1.433802505903950308 ) ) ;
#2720=CARTESIAN_POINT ( 'NONE',  ( -20.62524821624488069, -39.20140427513058512, 1.538452329860250378 ) ) ;
#2724=CARTESIAN_POINT ( 'NONE',  ( -31.61762450863942320, -48.95140427513057091, 9.857197362228843573 ) ) ;
#2731=CARTESIAN_POINT ( 'NONE',  ( -33.81171626276147890, -33.09859572486943335, 7.597606577763319713 ) ) ;
#2732=CARTESIAN_POINT ( 'NONE',  ( -20.61696076434619584, -31.20000000000000639, 1.486127417882100676 ) ) ;
#2739=CARTESIAN_POINT ( 'NONE',  ( -36.71751442127229836, -45.00000000000000711, -6.717514421272142044 ) ) ;
#2743=CARTESIAN_POINT ( 'NONE',  ( -25.99212434019154472, -45.65140427513058086, 7.988596311142242890 ) ) ;
#2747=CARTESIAN_POINT ( 'NONE',  ( -31.39812190974910422, -49.95000000000000995, 8.827394325379140483 ) ) ;
#2754=CARTESIAN_POINT ( 'NONE',  ( -20.13408869516453947, -43.04999999999999005, -1.562606840307983136 ) ) ;
#2755=CARTESIAN_POINT ( 'NONE',  ( -35.97294713907137975, -47.00140427513058938, -6.047868141099968398 ) ) ;
#2758=CARTESIAN_POINT ( 'NONE',  ( -39.85719736222883824, -42.54859572486944330, 1.617624508639602388 ) ) ;
#2765=CARTESIAN_POINT ( 'NONE',  ( -31.38201786482021305, -31.29859572486943975, -8.387063443159975762 ) ) ;
#2766=CARTESIAN_POINT ( 'NONE',  ( -20.14280263777121149, -41.04859572486944330, -1.617624508639600833 ) ) ;
#2767=CARTESIAN_POINT ( 'NONE',  ( -34.36011273255026310, -46.10140427513058370, 8.440510857627391061 ) ) ;
#2770=CARTESIAN_POINT ( 'NONE',  ( -34.48522952044771017, -44.15140427513058086, -8.925456012876139766 ) ) ;
#2780=CARTESIAN_POINT ( 'NONE',  ( -26.18828373723858149, -34.59859572486944046, -7.597606577763319713 ) ) ;
#2781=CARTESIAN_POINT ( 'NONE',  ( -28.51387258211773812, -37.80000000000000426, 9.383039235653802379 ) ) ;
#2786=CARTESIAN_POINT ( 'NONE',  ( -25.46513832392765408, -49.64999999999999147, 8.900167166472096270 ) ) ;
#2790=CARTESIAN_POINT ( 'NONE',  ( -25.99212434019154472, -39.65140427513058086, 7.988596311142242890 ) ) ;
#2793=CARTESIAN_POINT ( 'NONE',  ( -21.60464910494133406, -43.20000000000000995, 1.329692952841886155 ) ) ;
#2796=CARTESIAN_POINT ( 'NONE',  ( -31.56260684030781505, -46.94999999999998863, 9.865911304835510265 ) ) ;
#2797=CARTESIAN_POINT ( 'NONE',  ( -37.59760657776328685, -46.40140427513058086, 3.811716262761598362 ) ) ;
#2800=CARTESIAN_POINT ( 'NONE',  ( -20.14280263777121149, -47.04859572486944330, -1.617624508639600833 ) ) ;
#2802=CARTESIAN_POINT ( 'NONE',  ( -25.46513832392766119, -34.64999999999999858, 8.900167166472096270 ) ) ;
#2807=CARTESIAN_POINT ( 'NONE',  ( -28.65689575858256077, -34.44859572486944188, -8.836108267985801845 ) ) ;
#2808=CARTESIAN_POINT ( 'NONE',  ( -28.49241082802385350, -43.44859572486944188, -9.874625247442173404 ) ) ;
#2809=CARTESIAN_POINT ( 'NONE',  ( -21.51138689804841420, -41.90140427513058086, -4.265706762501151772 ) ) ;
#2814=FACE_OUTER_BOUND ( 'NONE', #6733, .T. ) ;
#2817=CARTESIAN_POINT ( 'NONE',  ( -36.36396103067902175, -30.00000000000000711, -6.363961030678874309 ) ) ;
#2820=CARTESIAN_POINT ( 'NONE',  ( -31.34310424141748896, -32.94859572486944188, 8.836108267985801845 ) ) ;
#2821=CARTESIAN_POINT ( 'NONE',  ( -20.61696076434619584, -34.20000000000000995, 1.486127417882100676 ) ) ;
#2823=CARTESIAN_POINT ( 'NONE',  ( -21.09983283352784156, -46.34999999999998721, 4.534861676072186043 ) ) ;
#2827=CARTESIAN_POINT ( 'NONE',  ( -28.51387258211773812, -49.80000000000001137, 9.383039235653802379 ) ) ;
#2829=CARTESIAN_POINT ( 'NONE',  ( -35.97294713907137975, -47.00140427513058938, -6.047868141099968398 ) ) ;
#2834=CARTESIAN_POINT ( 'NONE',  ( -37.57355545560112375, -41.40000000000000568, 3.858919247786223305 ) ) ;
#2841=CARTESIAN_POINT ( 'NONE',  ( -26.14108075221394856, -36.60000000000000853, -7.573555455601170827 ) ) ;
#2844=CARTESIAN_POINT ( 'NONE',  ( -38.92545601287626056, -48.84859572486942625, -4.485229520447501450 ) ) ;
#2851=CARTESIAN_POINT ( 'NONE',  ( -37.98859631114233792, -36.84859572486944046, -4.007875659808334490 ) ) ;
#2852=CARTESIAN_POINT ( 'NONE',  ( -39.85719736222883824, -36.54859572486943620, 1.617624508639602388 ) ) ;
#2853=CARTESIAN_POINT ( 'NONE',  ( -38.87487832006816291, -43.85140427513058370, -4.584493831696867971 ) ) ;
#2855=ORIENTED_EDGE ( 'NONE', *, *, #926, .F. ) ;
#2865=CARTESIAN_POINT ( 'NONE',  ( -23.95213185889994989, -32.49859572486943904, 5.972947139071243861 ) ) ;
#2866=CARTESIAN_POINT ( 'NONE',  ( -34.31290974752564438, -32.10000000000000142, 8.464561979789547053 ) ) ;
#2870=CARTESIAN_POINT ( 'NONE',  ( -36.71751442127229836, -48.00000000000000711, -6.717514421272142044 ) ) ;
#2877=CARTESIAN_POINT ( 'NONE',  ( -34.00787565980851213, -44.15140427513058086, -7.988596311142238449 ) ) ;
#2880=CARTESIAN_POINT ( 'NONE',  ( -21.17260567462091103, -49.05000000000000426, -1.398121909749241887 ) ) ;
#2886=PRODUCT_CONTEXT ( 'NONE', #5770, 'mechanical' ) ;
#2888=CARTESIAN_POINT ( 'NONE',  ( -34.05750781543318340, -39.14999999999999147, -7.963307464738195840 ) ) ;
#2891=CARTESIAN_POINT ( 'NONE',  ( -38.92545601287626056, -45.84859572486944046, -4.485229520447501450 ) ) ;
#2893=CARTESIAN_POINT ( 'NONE',  ( -39.86591130483550671, -35.55000000000000426, 1.562606840307984690 ) ) ;
#2897=DIRECTION ( 'NONE',  ( 0.7071067811865556774, 0.000000000000000000, 0.7071067811865393571 ) ) ;
#2899=CARTESIAN_POINT ( 'NONE',  ( -34.10713997105786888, -40.14859572486943762, -7.938018618334151455 ) ) ;
#2900=CARTESIAN_POINT ( 'NONE',  ( -23.28248557872775137, -31.50000000000000711, 6.717514421272141156 ) ) ;
#2901=CARTESIAN_POINT ( 'NONE',  ( -35.97294713907137975, -29.00140427513058583, -6.047868141099968398 ) ) ;
#2911=CARTESIAN_POINT ( 'NONE',  ( -38.40363834695740053, -39.69859572486944188, -1.277368040863739118 ) ) ;
#2912=CARTESIAN_POINT ( 'NONE',  ( -25.68709025247441602, -45.60000000000000853, -8.464561979789547053 ) ) ;
#2914=CARTESIAN_POINT ( 'NONE',  ( -34.31290974752564438, -47.10000000000000142, 8.464561979789547053 ) ) ;
#2922=CARTESIAN_POINT ( 'NONE',  ( -25.99212434019154472, -42.65140427513058086, 7.988596311142242890 ) ) ;
#2925=CARTESIAN_POINT ( 'NONE',  ( -38.39535089505872634, -44.70000000000000284, -1.329692952841885267 ) ) ;
#2929=CARTESIAN_POINT ( 'NONE',  ( -33.85891924778610473, -38.10000000000000853, 7.573555455601171715 ) ) ;
#2933=CARTESIAN_POINT ( 'NONE',  ( -31.48612741788231517, -30.30000000000000782, -9.383039235653804155 ) ) ;
#2935=CARTESIAN_POINT ( 'NONE',  ( -23.28248557872775137, -37.50000000000000711, 6.717514421272141156 ) ) ;
#2938=FACE_OUTER_BOUND ( 'NONE', #4171, .T. ) ;
#2940=CARTESIAN_POINT ( 'NONE',  ( -23.95213185889994989, -41.49859572486943904, 5.972947139071243861 ) ) ;
#2941=CARTESIAN_POINT ( 'NONE',  ( -38.44051085762733777, -45.39859572486944472, 4.360112732550414982 ) ) ;
#2942=CARTESIAN_POINT ( 'NONE',  ( -36.68005392025794009, -50.00140427513058938, -6.754974922286504757 ) ) ;
#2953=CARTESIAN_POINT ( 'NONE',  ( -36.04786814110010340, -36.99859572486943193, -5.972947139071243861 ) ) ;
#2954=CARTESIAN_POINT ( 'NONE',  ( -31.56260684030781505, -40.95000000000000995, 9.865911304835510265 ) ) ;
#2956=CARTESIAN_POINT ( 'NONE',  ( -31.43380250590416125, -29.30140427513058299, -9.391326687552492558 ) ) ;
#2965=CARTESIAN_POINT ( 'NONE',  ( -33.85891924778610473, -32.10000000000000142, 7.573555455601171715 ) ) ;
#2972=CARTESIAN_POINT ( 'NONE',  ( -38.39535089505872634, -41.70000000000000995, -1.329692952841885267 ) ) ;
#2976=CARTESIAN_POINT ( 'NONE',  ( -39.86591130483550671, -35.55000000000001137, 1.562606840307984468 ) ) ;
#2979=CARTESIAN_POINT ( 'NONE',  ( -34.31290974752564438, -44.10000000000000853, 8.464561979789547053 ) ) ;
#2984=CARTESIAN_POINT ( 'NONE',  ( -31.34310424141748896, -38.94859572486943478, 8.836108267985801845 ) ) ;
#2985=CARTESIAN_POINT ( 'NONE',  ( -36.75497492228666374, -48.99859572486944614, -6.680053920257780220 ) ) ;
#2986=CARTESIAN_POINT ( 'NONE',  ( -31.45313957808072303, -30.95140427513058157, 8.818680382772479120 ) ) ;
#2987=( GEOMETRIC_REPRESENTATION_CONTEXT ( 3 ) GLOBAL_UNCERTAINTY_ASSIGNED_CONTEXT ( ( #6434 ) ) GLOBAL_UNIT_ASSIGNED_CONTEXT ( ( #6932, #6316, #1111 ) ) REPRESENTATION_CONTEXT ( 'NONE', 'WORKASPACE' ) );
#2989=CARTESIAN_POINT ( 'NONE',  ( -20.61696076434619584, -31.20000000000000639, 1.486127417882100676 ) ) ;
#2996=CARTESIAN_POINT ( 'NONE',  ( -22.01140368885771892, -44.34859572486944046, 4.007875659808335378 ) ) ;
#2997=CARTESIAN_POINT ( 'NONE',  ( -21.53543802021056663, -39.90000000000000568, -4.312909747525783821 ) ) ;
#3001=CARTESIAN_POINT ( 'NONE',  ( -38.90016716647221529, -44.85000000000001563, -4.534861676072185155 ) ) ;
#3008=CARTESIAN_POINT ( 'NONE',  ( -36.01040764008574513, -33.00000000000000711, -6.010407640085605685 ) ) ;
#3016=ADVANCED_FACE ( 'NONE', ( #2814 ), #6195, .T. ) ;
#3018=CARTESIAN_POINT ( 'NONE',  ( -34.05750781543318340, -36.15000000000001279, -7.963307464738195840 ) ) ;
#3022=CARTESIAN_POINT ( 'NONE',  ( -26.14108075221394856, -30.60000000000000142, -7.573555455601170827 ) ) ;
#3023=CARTESIAN_POINT ( 'NONE',  ( -28.51387258211773812, -34.80000000000000426, 9.383039235653802379 ) ) ;
#3026=CARTESIAN_POINT ( 'NONE',  ( -38.90016716647221529, -44.85000000000000853, -4.534861676072185155 ) ) ;
#3027=SURFACE_STYLE_USAGE ( .BOTH. , #7067 ) ;
#3030=CARTESIAN_POINT ( 'NONE',  ( -22.45049566656107842, -34.89859572486943762, -3.906122232810846917 ) ) ;
#3031=CARTESIAN_POINT ( 'NONE',  ( -36.75497492228666374, -51.99859572486943193, -6.680053920257780220 ) ) ;
#3032=CARTESIAN_POINT ( 'NONE',  ( -22.40239342223677355, -32.90140427513058086, -3.811716262761597473 ) ) ;
#3035=CARTESIAN_POINT ( 'NONE',  ( -36.71751442127229836, -36.00000000000000711, -6.717514421272142044 ) ) ;
#3041=CARTESIAN_POINT ( 'NONE',  ( -28.61798213517984024, -38.79859572486943620, 8.387063443159973986 ) ) ;
#3042=CARTESIAN_POINT ( 'NONE',  ( -37.06321265474346660, -47.25000000000000711, 7.063212654743582952 ) ) ;
#3045=CARTESIAN_POINT ( 'NONE',  ( -28.56619749409589204, -39.80140427513057944, 9.391326687552490782 ) ) ;
#3053=CARTESIAN_POINT ( 'NONE',  ( -34.05750781543318340, -36.15000000000001279, -7.963307464738195840 ) ) ;
#3060=CARTESIAN_POINT ( 'NONE',  ( -37.57355545560112375, -44.40000000000000568, 3.858919247786223305 ) ) ;
#3065=CARTESIAN_POINT ( 'NONE',  ( -36.71751442127229836, -39.00000000000000711, -6.717514421272142044 ) ) ;
#3067=CARTESIAN_POINT ( 'NONE',  ( -34.53486167607238855, -36.15000000000000568, -8.900167166472096270 ) ) ;
#3070=CARTESIAN_POINT ( 'NONE',  ( -25.89286002894218086, -44.64859572486944472, 7.938018618334153231 ) ) ;
#3071=CARTESIAN_POINT ( 'NONE',  ( -31.50758917197619979, -44.94859572486942767, 9.874625247442176956 ) ) ;
#3072=CARTESIAN_POINT ( 'NONE',  ( -39.37475178375516549, -49.70140427513058512, -1.538452329860249712 ) ) ;
#3076=CARTESIAN_POINT ( 'NONE',  ( -20.13408869516453947, -37.05000000000001137, -1.562606840307983136 ) ) ;
#3082=CARTESIAN_POINT ( 'NONE',  ( -38.81868038277247734, -45.54859572486944330, 1.453139578080855365 ) ) ;
#3083=CARTESIAN_POINT ( 'NONE',  ( -25.68709025247441602, -48.60000000000000142, -8.464561979789547053 ) ) ;
#3085=CARTESIAN_POINT ( 'NONE',  ( -23.31994607974211675, -33.50140427513058228, 6.754974922286503869 ) ) ;
#3092=CARTESIAN_POINT ( 'NONE',  ( -35.97294713907137975, -50.00140427513058938, -6.047868141099968398 ) ) ;
#3104=CARTESIAN_POINT ( 'NONE',  ( -20.61696076434619584, -43.20000000000000995, 1.486127417882100676 ) ) ;
#3108=CARTESIAN_POINT ( 'NONE',  ( -31.34310424141748896, -44.94859572486942767, 8.836108267985801845 ) ) ;
#3109=CARTESIAN_POINT ( 'NONE',  ( -21.09983283352784156, -34.35000000000000853, 4.534861676072186043 ) ) ;
#3110=CARTESIAN_POINT ( 'NONE',  ( -26.09387776718931917, -35.60140427513057659, -7.549504333439021941 ) ) ;
#3111=AXIS2_PLACEMENT_3D ( 'NONE', #4780, #6186, #2231 ) ;
#3117=CARTESIAN_POINT ( 'NONE',  ( -34.31290974752564438, -35.10000000000000853, 8.464561979789547053 ) ) ;
#3123=CARTESIAN_POINT ( 'NONE',  ( -25.41550616830297571, -32.64859572486943762, 8.874878320068054549 ) ) ;
#3124=CARTESIAN_POINT ( 'NONE',  ( -23.31994607974211675, -30.50140427513058583, 6.754974922286503869 ) ) ;
#3128=CARTESIAN_POINT ( 'NONE',  ( -34.36011273255026310, -40.10140427513057659, 8.440510857627391061 ) ) ;
#3137=CARTESIAN_POINT ( 'NONE',  ( -23.68028341417693738, -33.75000000000001421, -6.319716585823198507 ) ) ;
#3139=CARTESIAN_POINT ( 'NONE',  ( -25.99212434019154472, -30.65140427513057730, 7.988596311142242890 ) ) ;
#3153=CARTESIAN_POINT ( 'NONE',  ( -39.86591130483550671, -47.55000000000000426, 1.562606840307984690 ) ) ;
#3157=CARTESIAN_POINT ( 'NONE',  ( -22.45049566656107842, -49.89859572486943762, -3.906122232810846917 ) ) ;
#3158=CARTESIAN_POINT ( 'NONE',  ( -20.13408869516453947, -34.04999999999998295, -1.562606840307983136 ) ) ;
#3159=CARTESIAN_POINT ( 'NONE',  ( -25.99212434019154472, -36.65140427513058086, 7.988596311142242890 ) ) ;
#3163=CARTESIAN_POINT ( 'NONE',  ( -23.24502507771338600, -35.49859572486943193, 6.680053920257780220 ) ) ;
#3164=CARTESIAN_POINT ( 'NONE',  ( -22.93678734525658314, -33.75000000000001421, -7.063212654743582952 ) ) ;
#3169=CARTESIAN_POINT ( 'NONE',  ( -22.97617564697422665, -31.74859572486943193, -7.102600956461224690 ) ) ;
#3170=CARTESIAN_POINT ( 'NONE',  ( -28.38237549136062654, -32.45140427513058512, -9.857197362228843573 ) ) ;
#3172=CARTESIAN_POINT ( 'NONE',  ( -23.31994607974211675, -36.50140427513057517, 6.754974922286503869 ) ) ;
#3179=CARTESIAN_POINT ( 'NONE',  ( -28.60187809025093841, -42.44999999999999574, -8.827394325379140483 ) ) ;
#3184=CARTESIAN_POINT ( 'NONE',  ( -34.00787565980851213, -35.15140427513058086, -7.988596311142238449 ) ) ;
#3188=CARTESIAN_POINT ( 'NONE',  ( -31.32969295284206979, -39.30000000000001137, -8.395350895058669494 ) ) ;
#3190=CARTESIAN_POINT ( 'NONE',  ( -39.38303923565386100, -50.70000000000000995, -1.486127417882099788 ) ) ;
#3193=CARTESIAN_POINT ( 'NONE',  ( -33.81171626276147890, -48.09859572486944046, 7.597606577763319713 ) ) ;
#3194=CARTESIAN_POINT ( 'NONE',  ( -34.53486167607238144, -39.14999999999999147, -8.900167166472096270 ) ) ;
#3195=CARTESIAN_POINT ( 'NONE',  ( -38.38706344316003793, -40.70140427513058512, -1.382017864820032083 ) ) ;
#3198=MECHANICAL_DESIGN_GEOMETRIC_PRESENTATION_REPRESENTATION('',(#4896),#6085);
#3200=CARTESIAN_POINT ( 'NONE',  ( -20.14280263777121149, -41.04859572486944330, -1.617624508639600833 ) ) ;
#3201=CARTESIAN_POINT ( 'NONE',  ( -21.53543802021056663, -39.90000000000000568, -4.312909747525783821 ) ) ;
#3207=CARTESIAN_POINT ( 'NONE',  ( -38.44051085762733777, -33.39859572486943762, 4.360112732550414982 ) ) ;
#3208=CARTESIAN_POINT ( 'NONE',  ( -37.10260095646111012, -34.25140427513057517, 7.023824353025939438 ) ) ;
#3212=CARTESIAN_POINT ( 'NONE',  ( -25.51477047955235378, -36.65140427513058086, 8.925456012876139766 ) ) ;
#3220=CARTESIAN_POINT ( 'NONE',  ( -22.03669253526174998, -40.35000000000000142, 4.057507815433014642 ) ) ;
#3225=CARTESIAN_POINT ( 'NONE',  ( -39.38303923565386100, -32.70000000000000995, -1.486127417882099788 ) ) ;
#3227=CARTESIAN_POINT ( 'NONE',  ( -37.93801861833426159, -34.85140427513057659, -4.107139971057695682 ) ) ;
#3229=CARTESIAN_POINT ( 'NONE',  ( -26.14108075221394856, -33.60000000000000142, -7.573555455601170827 ) ) ;
#3232=CARTESIAN_POINT ( 'NONE',  ( -20.61696076434619584, -46.20000000000000284, 1.486127417882100676 ) ) ;
#3235=CARTESIAN_POINT ( 'NONE',  ( -22.01140368885771892, -50.34859572486944046, 4.007875659808335378 ) ) ;
#3236=CARTESIAN_POINT ( 'NONE',  ( -20.13408869516453947, -40.05000000000001137, -1.562606840307983136 ) ) ;
#3237=CARTESIAN_POINT ( 'NONE',  ( -25.99212434019154472, -39.65140427513058086, 7.988596311142242890 ) ) ;
#3241=CARTESIAN_POINT ( 'NONE',  ( -34.26570676250101855, -42.09859572486944046, 8.488613101951703044 ) ) ;
#3242=CARTESIAN_POINT ( 'NONE',  ( -25.68709025247441602, -42.60000000000000853, -8.464561979789547053 ) ) ;
#3250=CARTESIAN_POINT ( 'NONE',  ( -37.98859631114233792, -48.84859572486942625, -4.007875659808334490 ) ) ;
#3251=CARTESIAN_POINT ( 'NONE',  ( -39.37475178375516549, -34.70140427513057091, -1.538452329860249712 ) ) ;
#3253=CARTESIAN_POINT ( 'NONE',  ( -34.36011273255026310, -43.10140427513058370, 8.440510857627391061 ) ) ;
#3261=CARTESIAN_POINT ( 'NONE',  ( -31.39812190974910422, -37.94999999999998153, 8.827394325379140483 ) ) ;
#3267=CARTESIAN_POINT ( 'NONE',  ( -28.43739315969223824, -42.44999999999999574, -9.865911304835512041 ) ) ;
#3270=CARTESIAN_POINT ( 'NONE',  ( -35.97294713907137975, -38.00140427513057517, -6.047868141099968398 ) ) ;
#3275=CARTESIAN_POINT ( 'NONE',  ( -28.60187809025093841, -36.44999999999999574, -8.827394325379140483 ) ) ;
#3278=CARTESIAN_POINT ( 'NONE',  ( -23.28248557872775137, -49.50000000000000711, 6.717514421272141156 ) ) ;
#3282=CARTESIAN_POINT ( 'NONE',  ( -22.93678734525658314, -33.75000000000001421, -7.063212654743582952 ) ) ;
#3284=CARTESIAN_POINT ( 'NONE',  ( -24.02705286092866643, -36.50140427513057517, 6.047868141099968398 ) ) ;
#3289=CARTESIAN_POINT ( 'NONE',  ( -38.92545601287626056, -33.84859572486942625, -4.485229520447501450 ) ) ;
#3298=CARTESIAN_POINT ( 'NONE',  ( -26.18828373723858149, -31.59859572486943335, -7.597606577763319713 ) ) ;
#3299=CARTESIAN_POINT ( 'NONE',  ( -31.50758917197619979, -32.94859572486944188, 9.874625247442176956 ) ) ;
#3300=CARTESIAN_POINT ( 'NONE',  ( -31.43380250590416125, -32.30140427513056522, -9.391326687552492558 ) ) ;
#3302=CARTESIAN_POINT ( 'NONE',  ( -31.43380250590416125, -41.30140427513058654, -9.391326687552492558 ) ) ;
#3310=CARTESIAN_POINT ( 'NONE',  ( -26.14108075221394856, -45.60000000000000853, -7.573555455601170827 ) ) ;
#3315=CARTESIAN_POINT ( 'NONE',  ( -34.31290974752564438, -44.10000000000000853, 8.464561979789547053 ) ) ;
#3318=CARTESIAN_POINT ( 'NONE',  ( -21.16389173201424612, -30.05140427513057944, -1.343104241417630185 ) ) ;
#3321=CARTESIAN_POINT ( 'NONE',  ( -21.17260567462091103, -31.05000000000000426, -1.398121909749241887 ) ) ;
#3324=CARTESIAN_POINT ( 'NONE',  ( -36.71751442127229836, -51.00000000000000711, -6.717514421272142044 ) ) ;
#3327=CARTESIAN_POINT ( 'NONE',  ( -39.86591130483550671, -44.55000000000001137, 1.562606840307984468 ) ) ;
#3328=CARTESIAN_POINT ( 'NONE',  ( -25.99212434019154472, -48.65140427513057375, 7.988596311142242890 ) ) ;
#3330=CARTESIAN_POINT ( 'NONE',  ( -31.53845232986046554, -37.29859572486943620, -9.374751783755117529 ) ) ;
#3337=CARTESIAN_POINT ( 'NONE',  ( -28.67030704715798350, -49.80000000000001137, 8.395350895058669494 ) ) ;
#3338=CARTESIAN_POINT ( 'NONE',  ( -23.24502507771338600, -38.49859572486943904, 6.680053920257780220 ) ) ;
#3339=CARTESIAN_POINT ( 'NONE',  ( -31.61762450863942320, -36.95140427513057801, 9.857197362228843573 ) ) ;
#3343=CARTESIAN_POINT ( 'NONE',  ( -34.48522952044771017, -47.15140427513058086, -8.925456012876139766 ) ) ;
#3352=CARTESIAN_POINT ( 'NONE',  ( -23.98959235991431171, -46.50000000000000711, 6.010407640085604797 ) ) ;
#3353=CARTESIAN_POINT ( 'NONE',  ( -20.13408869516453947, -34.04999999999998295, -1.562606840307983136 ) ) ;
#3358=CARTESIAN_POINT ( 'NONE',  ( -23.28248557872775137, -43.50000000000001421, 6.717514421272141156 ) ) ;
#3362=CARTESIAN_POINT ( 'NONE',  ( -37.59760657776328685, -34.40140427513058086, 3.811716262761598362 ) ) ;
#3364=CARTESIAN_POINT ( 'NONE',  ( -38.39535089505872634, -35.70000000000000995, -1.329692952841885267 ) ) ;
#3370=CARTESIAN_POINT ( 'NONE',  ( -38.46456197978948666, -44.40000000000000568, 4.312909747525784709 ) ) ;
#3371=CARTESIAN_POINT ( 'NONE',  ( -23.64089511245930098, -47.75140427513058938, -6.280328284105564762 ) ) ;
#3374=CARTESIAN_POINT ( 'NONE',  ( -25.73429323749904185, -46.59859572486944046, -8.488613101951701267 ) ) ;
#3381=CARTESIAN_POINT ( 'NONE',  ( -23.71967171589458445, -31.74859572486943193, -6.359104887540838469 ) ) ;
#3382=CARTESIAN_POINT ( 'NONE',  ( -21.07454398712378918, -41.34859572486944757, 4.485229520447505003 ) ) ;
#3383=CARTESIAN_POINT ( 'NONE',  ( -37.10260095646111012, -37.25140427513058228, 7.023824353025939438 ) ) ;
#3387=CARTESIAN_POINT ( 'NONE',  ( -31.43380250590416125, -47.30140427513057944, -9.391326687552492558 ) ) ;
#3396=CARTESIAN_POINT ( 'NONE',  ( -21.59636165304264921, -35.19859572486944188, 1.277368040863740228 ) ) ;
#3397=CARTESIAN_POINT ( 'NONE',  ( -34.31290974752564438, -38.10000000000000853, 8.464561979789547053 ) ) ;
#3401=CARTESIAN_POINT ( 'NONE',  ( -39.86591130483550671, -44.55000000000001137, 1.562606840307984468 ) ) ;
#3403=EDGE_CURVE ( 'NONE', #8652, #7915, #8265, .T. ) ;
#3404=CARTESIAN_POINT ( 'NONE',  ( -38.83610826798580717, -40.55140427513058654, 1.343104241417631073 ) ) ;
#3405=COLOUR_RGB ( '', 0.08235294, 0.09019608, 0.10196078) ;
#3407=CARTESIAN_POINT ( 'NONE',  ( -22.03669253526174998, -46.34999999999999432, 4.057507815433014642 ) ) ;
#3414=CARTESIAN_POINT ( 'NONE',  ( -23.28248557872775137, -46.50000000000000711, 6.717514421272141156 ) ) ;
#3415=CARTESIAN_POINT ( 'NONE',  ( -36.01040764008574513, -30.00000000000000711, -6.010407640085605685 ) ) ;
#3420=CARTESIAN_POINT ( 'NONE',  ( -28.46154767013959486, -50.79859572486945041, 9.374751783755112200 ) ) ;
#3422=CARTESIAN_POINT ( 'NONE',  ( -25.68709025247441602, -33.60000000000000142, -8.464561979789547053 ) ) ;
#3427=CARTESIAN_POINT ( 'NONE',  ( -36.04786814110010340, -30.99859572486944259, -5.972947139071243861 ) ) ;
#3428=CARTESIAN_POINT ( 'NONE',  ( -38.92545601287626056, -39.84859572486944046, -4.485229520447501450 ) ) ;
#3429=CARTESIAN_POINT ( 'NONE',  ( -20.62524821624488069, -42.20140427513058512, 1.538452329860250378 ) ) ;
#3432=CARTESIAN_POINT ( 'NONE',  ( -38.87487832006816291, -40.85140427513057659, -4.584493831696867971 ) ) ;
#3440=CARTESIAN_POINT ( 'NONE',  ( -21.18131961722757595, -32.04859572486944330, -1.453139578080854699 ) ) ;
#3441=CARTESIAN_POINT ( 'NONE',  ( -39.38303923565386100, -38.70000000000000284, -1.486127417882099788 ) ) ;
#3447=CARTESIAN_POINT ( 'NONE',  ( -38.90016716647221529, -47.85000000000000853, -4.534861676072185155 ) ) ;
#3449=CARTESIAN_POINT ( 'NONE',  ( -22.40239342223677355, -47.90140427513058086, -3.811716262761597473 ) ) ;
#3454=CARTESIAN_POINT ( 'NONE',  ( -26.14108075221394856, -48.60000000000000142, -7.573555455601170827 ) ) ;
#3459=CARTESIAN_POINT ( 'NONE',  ( -34.31290974752564438, -50.10000000000000853, 8.464561979789547053 ) ) ;
#3460=CARTESIAN_POINT ( 'NONE',  ( -23.98959235991431171, -31.50000000000000711, 6.010407640085604797 ) ) ;
#3463=CARTESIAN_POINT ( 'NONE',  ( -21.55948914237271907, -46.89859572486944472, -4.360112732550413206 ) ) ;
#3465=CARTESIAN_POINT ( 'NONE',  ( -25.68709025247441602, -30.60000000000000142, -8.464561979789547053 ) ) ;
#3470=CARTESIAN_POINT ( 'NONE',  ( -31.38201786482021305, -34.29859572486943620, -8.387063443159975762 ) ) ;
#3471=CARTESIAN_POINT ( 'NONE',  ( -36.75497492228666374, -42.99859572486943904, -6.680053920257780220 ) ) ;
#3472=CARTESIAN_POINT ( 'NONE',  ( -38.48861310195163554, -40.40140427513058086, 4.265706762501153548 ) ) ;
#3483=CARTESIAN_POINT ( 'NONE',  ( -23.95213185889994989, -35.49859572486943193, 5.972947139071243861 ) ) ;
#3484=CARTESIAN_POINT ( 'NONE',  ( -28.51387258211773812, -34.80000000000000426, 9.383039235653802379 ) ) ;
#3487=CARTESIAN_POINT ( 'NONE',  ( -31.56260684030781505, -46.94999999999998863, 9.865911304835510265 ) ) ;
#3490=CARTESIAN_POINT ( 'NONE',  ( -39.86591130483550671, -50.55000000000001137, 1.562606840307984468 ) ) ;
#3493=CARTESIAN_POINT ( 'NONE',  ( -28.72263195913613387, -45.80140427513057944, 8.403638346957361449 ) ) ;
#3497=CARTESIAN_POINT ( 'NONE',  ( -38.82739432537914581, -47.55000000000000426, 1.398121909749243663 ) ) ;
#3502=SURFACE_STYLE_USAGE ( .BOTH. , #8347 ) ;
#3503=CARTESIAN_POINT ( 'NONE',  ( -38.90016716647221529, -50.84999999999999432, -4.534861676072185155 ) ) ;
#3504=CARTESIAN_POINT ( 'NONE',  ( -21.17260567462091458, -37.05000000000001137, -1.398121909749242331 ) ) ;
#3508=CARTESIAN_POINT ( 'NONE',  ( -34.58449383169706692, -43.14859572486943762, -8.874878320068054549 ) ) ;
#3514=CARTESIAN_POINT ( 'NONE',  ( -33.81171626276147890, -36.09859572486943335, 7.597606577763319713 ) ) ;
#3515=CARTESIAN_POINT ( 'NONE',  ( -20.60867331244750034, -44.19859572486944899, 1.433802505903951419 ) ) ;
#3516=CARTESIAN_POINT ( 'NONE',  ( -25.51477047955235378, -42.65140427513058086, 8.925456012876139766 ) ) ;
#3524=ORIENTED_EDGE ( 'NONE', *, *, #926, .T. ) ;
#3525=CARTESIAN_POINT ( 'NONE',  ( -21.60464910494133406, -49.20000000000000995, 1.329692952841886155 ) ) ;
#3526=CARTESIAN_POINT ( 'NONE',  ( -21.53543802021056663, -30.90000000000000924, -4.312909747525783821 ) ) ;
#3528=CARTESIAN_POINT ( 'NONE',  ( -39.38303923565386100, -44.70000000000000284, -1.486127417882099788 ) ) ;
#3535=CARTESIAN_POINT ( 'NONE',  ( -36.35910488754074521, -43.25140427513058228, 6.280328284105565650 ) ) ;
#3540=CARTESIAN_POINT ( 'NONE',  ( -25.94249218456686279, -46.65000000000001279, 7.963307464738194952 ) ) ;
#3544=CARTESIAN_POINT ( 'NONE',  ( -28.60187809025093841, -42.44999999999999574, -8.827394325379140483 ) ) ;
#3547=CARTESIAN_POINT ( 'NONE',  ( -39.85719736222883824, -48.54859572486944330, 1.617624508639602388 ) ) ;
#3553=CARTESIAN_POINT ( 'NONE',  ( -25.89286002894218086, -38.64859572486943762, 7.938018618334153231 ) ) ;
#3554=CARTESIAN_POINT ( 'NONE',  ( -34.53486167607238144, -30.15000000000000213, -8.900167166472096270 ) ) ;
#3555=CARTESIAN_POINT ( 'NONE',  ( -22.06198138166579170, -30.35140427513058015, 4.107139971057695682 ) ) ;
#3566=EDGE_LOOP ( 'NONE', ( #6019, #2855 ) ) ;
#3567=CARTESIAN_POINT ( 'NONE',  ( -25.94249218456686279, -49.64999999999999147, 7.963307464738195840 ) ) ;
#3568=CARTESIAN_POINT ( 'NONE',  ( -25.68709025247441602, -39.60000000000000853, -8.464561979789547053 ) ) ;
#3572=CARTESIAN_POINT ( 'NONE',  ( -20.61696076434619584, -46.20000000000000284, 1.486127417882100676 ) ) ;
#3576=CARTESIAN_POINT ( 'NONE',  ( -21.09983283352784156, -49.35000000000000853, 4.534861676072186043 ) ) ;
#3580=CARTESIAN_POINT ( 'NONE',  ( -28.54686042191934092, -47.45140427513057091, -8.818680382772479120 ) ) ;
#3583=CARTESIAN_POINT ( 'NONE',  ( -25.94249218456686279, -49.64999999999999858, 7.963307464738194952 ) ) ;
#3587=FILL_AREA_STYLE_COLOUR ( '', #5729 ) ;
#3588=CARTESIAN_POINT ( 'NONE',  ( -31.39812190974910422, -40.95000000000000995, 8.827394325379140483 ) ) ;
#3592=CARTESIAN_POINT ( 'NONE',  ( -20.61696076434619584, -31.20000000000000639, 1.486127417882100676 ) ) ;
#3598=CARTESIAN_POINT ( 'NONE',  ( -26.18828373723858149, -40.59859572486944757, -7.597606577763319713 ) ) ;
#3599=CARTESIAN_POINT ( 'NONE',  ( -28.51387258211773812, -31.80000000000000782, 9.383039235653802379 ) ) ;
#3600=CARTESIAN_POINT ( 'NONE',  ( -25.51477047955235378, -48.65140427513057375, 8.925456012876139766 ) ) ;
#3608=CARTESIAN_POINT ( 'NONE',  ( -37.54950433343896776, -42.39859572486944472, 3.906122232810848249 ) ) ;
#3609=CARTESIAN_POINT ( 'NONE',  ( -38.46456197978948666, -44.40000000000000568, 4.312909747525784709 ) ) ;
#3612=CARTESIAN_POINT ( 'NONE',  ( -39.86591130483550671, -47.54999999999999716, 1.562606840307984468 ) ) ;
#3620=CARTESIAN_POINT ( 'NONE',  ( -38.39535089505872634, -32.70000000000000995, -1.329692952841885267 ) ) ;
#3628=CARTESIAN_POINT ( 'NONE',  ( -33.85891924778610473, -35.10000000000000853, 7.573555455601171715 ) ) ;
#3631=CARTESIAN_POINT ( 'NONE',  ( -28.43739315969223824, -36.45000000000000284, -9.865911304835512041 ) ) ;
#3633=CARTESIAN_POINT ( 'NONE',  ( -37.06321265474346660, -41.25000000000000711, 7.063212654743582952 ) ) ;
#3635=( NAMED_UNIT ( * ) SI_UNIT ( $, .STERADIAN. ) SOLID_ANGLE_UNIT ( ) );
#3639=CARTESIAN_POINT ( 'NONE',  ( -22.01140368885771892, -38.34859572486944046, 4.007875659808335378 ) ) ;
#3640=CARTESIAN_POINT ( 'NONE',  ( -21.55948914237271907, -49.89859572486943762, -4.360112732550413206 ) ) ;
#3641=CARTESIAN_POINT ( 'NONE',  ( -28.72263195913613387, -30.80140427513057233, 8.403638346957361449 ) ) ;
#3642=ADVANCED_FACE ( 'NONE', ( #2938 ), #7850, .F. ) ;
#3652=CARTESIAN_POINT ( 'NONE',  ( -26.18828373723858149, -43.59859572486944046, -7.597606577763319713 ) ) ;
#3653=CARTESIAN_POINT ( 'NONE',  ( -31.56260684030781505, -46.94999999999998863, 9.865911304835510265 ) ) ;
#3655=CARTESIAN_POINT ( 'NONE',  ( -20.62524821624488069, -30.20140427513057446, 1.538452329860250378 ) ) ;
#3656=CARTESIAN_POINT ( 'NONE',  ( -36.71751442127229836, -30.00000000000000711, -6.717514421272142044 ) ) ;
#3663=CARTESIAN_POINT ( 'NONE',  ( -21.17260567462091458, -31.05000000000000782, -1.398121909749242331 ) ) ;
#3670=CARTESIAN_POINT ( 'NONE',  ( -36.01040764008574513, -42.00000000000000711, -6.010407640085605685 ) ) ;
#3673=CARTESIAN_POINT ( 'NONE',  ( -34.05750781543319050, -30.15000000000000568, -7.963307464738194952 ) ) ;
#3674=CARTESIAN_POINT ( 'NONE',  ( -22.93678734525658314, -30.75000000000000000, -7.063212654743582952 ) ) ;
#3677=CARTESIAN_POINT ( 'NONE',  ( -25.46513832392766119, -43.64999999999999858, 8.900167166472096270 ) ) ;
#3681=CARTESIAN_POINT ( 'NONE',  ( -34.10713997105786888, -37.14859572486943762, -7.938018618334151455 ) ) ;
#3683=CARTESIAN_POINT ( 'NONE',  ( -23.24502507771338600, -50.49859572486944614, 6.680053920257780220 ) ) ;
#3684=CARTESIAN_POINT ( 'NONE',  ( -22.89739904353894318, -47.75140427513058938, -7.023824353025938549 ) ) ;
#3692=DIRECTION ( 'NONE',  ( 1.000000000000000000, 0.000000000000000000, 0.000000000000000000 ) ) ;
#3694=CARTESIAN_POINT ( 'NONE',  ( -36.04786814110010340, -42.99859572486943904, -5.972947139071243861 ) ) ;
#3695=CARTESIAN_POINT ( 'NONE',  ( -38.90016716647221529, -41.84999999999999432, -4.534861676072185155 ) ) ;
#3698=CARTESIAN_POINT ( 'NONE',  ( -21.51138689804841420, -38.90140427513058086, -4.265706762501151772 ) ) ;
#3706=CARTESIAN_POINT ( 'NONE',  ( -38.82739432537914581, -35.55000000000001137, 1.398121909749243441 ) ) ;
#3707=CIRCLE ( 'NONE', #4828, 0.5000000000000001110 ) ;
#3710=CARTESIAN_POINT ( 'NONE',  ( -37.57355545560112375, -50.40000000000000568, 3.858919247786223305 ) ) ;
#3713=CARTESIAN_POINT ( 'NONE',  ( -28.67030704715798350, -43.80000000000000426, 8.395350895058669494 ) ) ;
#3718=CARTESIAN_POINT ( 'NONE',  ( -39.86591130483550671, -38.54999999999999716, 1.562606840307984468 ) ) ;
#3721=CARTESIAN_POINT ( 'NONE',  ( -21.53543802021056663, -39.90000000000000568, -4.312909747525783821 ) ) ;
#3724=CARTESIAN_POINT ( 'NONE',  ( -23.95213185889994989, -44.49859572486944614, 5.972947139071243861 ) ) ;
#3725=CARTESIAN_POINT ( 'NONE',  ( -38.92545601287626056, -51.84859572486944757, -4.485229520447501450 ) ) ;
#3726=CARTESIAN_POINT ( 'NONE',  ( -38.48861310195163554, -49.40140427513058086, 4.265706762501153548 ) ) ;
#3730=CARTESIAN_POINT ( 'NONE',  ( -34.31290974752564438, -38.10000000000000853, 8.464561979789547053 ) ) ;
#3731=DIRECTION ( 'NONE',  ( -0.7061138087190628188, 0.05297714858780449426, 0.7061138087190792501 ) ) ;
#3736=CARTESIAN_POINT ( 'NONE',  ( -21.59636165304264921, -41.19859572486944188, 1.277368040863740228 ) ) ;
#3737=CARTESIAN_POINT ( 'NONE',  ( -31.48612741788231517, -48.30000000000001137, -9.383039235653804155 ) ) ;
#3739=CARTESIAN_POINT ( 'NONE',  ( -34.48522952044771017, -35.15140427513058086, -8.925456012876139766 ) ) ;
#3747=CARTESIAN_POINT ( 'NONE',  ( -23.98959235991431171, -37.50000000000000711, 6.010407640085604797 ) ) ;
#3761=CARTESIAN_POINT ( 'NONE',  ( -28.43739315969223824, -42.45000000000000284, -9.865911304835512041 ) ) ;
#3765=CARTESIAN_POINT ( 'NONE',  ( -22.01140368885771892, -44.34859572486944046, 4.007875659808335378 ) ) ;
#3767=CARTESIAN_POINT ( 'NONE',  ( -21.53543802021056663, -39.90000000000000568, -4.312909747525783821 ) ) ;
#3768=CARTESIAN_POINT ( 'NONE',  ( -22.06198138166579170, -42.35140427513057659, 4.107139971057695682 ) ) ;
#3773=CARTESIAN_POINT ( 'NONE',  ( -34.53486167607238144, -36.15000000000001279, -8.900167166472096270 ) ) ;
#3778=CARTESIAN_POINT ( 'NONE',  ( -36.01040764008574513, -51.00000000000000711, -6.010407640085605685 ) ) ;
#3782=CARTESIAN_POINT ( 'NONE',  ( -31.34310424141748896, -50.94859572486944899, 8.836108267985801845 ) ) ;
#3783=CARTESIAN_POINT ( 'NONE',  ( -22.89739904353894318, -29.75140427513057517, -7.023824353025938549 ) ) ;
#3785=CARTESIAN_POINT ( 'NONE',  ( -31.61762450863942320, -36.95140427513057801, 9.857197362228843573 ) ) ;
#3791=ORIENTED_EDGE ( 'NONE', *, *, #6970, .T. ) ;
#3792=CARTESIAN_POINT ( 'NONE',  ( -22.42644454439892598, -30.90000000000000924, -3.858919247786222861 ) ) ;
#3802=CARTESIAN_POINT ( 'NONE',  ( -38.46456197978948666, -50.40000000000000568, 4.312909747525784709 ) ) ;
#3805=CARTESIAN_POINT ( 'NONE',  ( -31.34310424141748896, -50.94859572486944899, 8.836108267985801845 ) ) ;
#3806=CARTESIAN_POINT ( 'NONE',  ( -37.06321265474346660, -32.25000000000000711, 7.063212654743582952 ) ) ;
#3807=CARTESIAN_POINT ( 'NONE',  ( -38.83610826798580717, -43.55140427513057944, 1.343104241417631073 ) ) ;
#3811=CARTESIAN_POINT ( 'NONE',  ( -22.97617564697422665, -34.74859572486943904, -7.102600956461224690 ) ) ;
#3812=CARTESIAN_POINT ( 'NONE',  ( -25.46513832392765408, -34.64999999999998437, 8.900167166472096270 ) ) ;
#3813=PRODUCT ( 'shock absorber', 'shock absorber', '', ( #2886 ) ) ;
#3819=CARTESIAN_POINT ( 'NONE',  ( -31.34310424141748896, -47.94859572486943478, 8.836108267985801845 ) ) ;
#3820=CARTESIAN_POINT ( 'NONE',  ( -21.51138689804841420, -29.90140427513058796, -4.265706762501151772 ) ) ;
#3824=CARTESIAN_POINT ( 'NONE',  ( -31.61762450863942320, -33.95140427513058512, 9.857197362228843573 ) ) ;
#3832=CARTESIAN_POINT ( 'NONE',  ( -38.82739432537914581, -41.55000000000001137, 1.398121909749243441 ) ) ;
#3837=CARTESIAN_POINT ( 'NONE',  ( -38.38706344316003793, -31.70140427513057091, -1.382017864820032083 ) ) ;
#3842=CARTESIAN_POINT ( 'NONE',  ( -37.96330746473829976, -32.85000000000000142, -4.057507815433013754 ) ) ;
#3848=CARTESIAN_POINT ( 'NONE',  ( -22.01140368885771892, -47.34859572486942625, 4.007875659808335378 ) ) ;
#3849=CARTESIAN_POINT ( 'NONE',  ( -34.31290974752564438, -38.10000000000000853, 8.464561979789547053 ) ) ;
#3850=CARTESIAN_POINT ( 'NONE',  ( -37.59760657776328685, -37.40140427513058796, 3.811716262761598362 ) ) ;
#3856=CARTESIAN_POINT ( 'NONE',  ( -21.55948914237271907, -34.89859572486943762, -4.360112732550413206 ) ) ;
#3857=CARTESIAN_POINT ( 'NONE',  ( -34.53486167607238144, -39.14999999999999147, -8.900167166472096270 ) ) ;
#3864=CARTESIAN_POINT ( 'NONE',  ( -22.45049566656107842, -49.89859572486943762, -3.906122232810846917 ) ) ;
#3866=CARTESIAN_POINT ( 'NONE',  ( -39.37475178375516549, -31.70140427513057091, -1.538452329860249712 ) ) ;
#3870=CARTESIAN_POINT ( 'NONE',  ( -38.48861310195163554, -37.40140427513058796, 4.265706762501153548 ) ) ;
#3877=CARTESIAN_POINT ( 'NONE',  ( -23.68028341417693738, -42.75000000000001421, -6.319716585823198507 ) ) ;
#3881=CARTESIAN_POINT ( 'NONE',  ( -34.31290974752564438, -38.10000000000000853, 8.464561979789547053 ) ) ;
#3883=CARTESIAN_POINT ( 'NONE',  ( -34.00787565980851213, -29.15140427513058441, -7.988596311142238449 ) ) ;
#3886=CARTESIAN_POINT ( 'NONE',  ( -22.03669253526174998, -37.35000000000000853, 4.057507815433014642 ) ) ;
#3892=CARTESIAN_POINT ( 'NONE',  ( -28.61798213517984024, -47.79859572486944330, 8.387063443159973986 ) ) ;
#3893=CARTESIAN_POINT ( 'NONE',  ( -21.09983283352784156, -37.35000000000000853, 4.534861676072186043 ) ) ;
#3894=CARTESIAN_POINT ( 'NONE',  ( -35.97294713907137975, -44.00140427513057517, -6.047868141099968398 ) ) ;
#3898=CARTESIAN_POINT ( 'NONE',  ( -39.39132668755255651, -36.69859572486944188, -1.433802505903950308 ) ) ;
#3899=CARTESIAN_POINT ( 'NONE',  ( -21.53543802021056663, -42.90000000000000568, -4.312909747525783821 ) ) ;
#3906=CARTESIAN_POINT ( 'NONE',  ( -26.18828373723858149, -46.59859572486944046, -7.597606577763319713 ) ) ;
#3907=CARTESIAN_POINT ( 'NONE',  ( -25.63988726744978663, -29.60140427513057659, -8.440510857627391061 ) ) ;
#3912=CARTESIAN_POINT ( 'NONE',  ( -21.12512167993187973, -42.35140427513057659, 4.584493831696868860 ) ) ;
#3915=CARTESIAN_POINT ( 'NONE',  ( -37.96330746473829976, -50.85000000000000142, -4.057507815433013754 ) ) ;
#3920=CARTESIAN_POINT ( 'NONE',  ( -28.60187809025093841, -45.45000000000000995, -8.827394325379140483 ) ) ;
#3925=CARTESIAN_POINT ( 'NONE',  ( -28.43739315969223824, -48.44999999999999574, -9.865911304835512041 ) ) ;
#3929=CARTESIAN_POINT ( 'NONE',  ( -23.64089511245930098, -35.75140427513057517, -6.280328284105564762 ) ) ;
#3931=CARTESIAN_POINT ( 'NONE',  ( -21.17260567462091103, -37.05000000000000426, -1.398121909749241887 ) ) ;
#3936=CARTESIAN_POINT ( 'NONE',  ( -37.06321265474346660, -35.24999999999998579, 7.063212654743582952 ) ) ;
#3937=CARTESIAN_POINT ( 'NONE',  ( -38.83610826798580717, -40.55140427513058654, 1.343104241417631073 ) ) ;
#3941=CARTESIAN_POINT ( 'NONE',  ( -39.85719736222883824, -39.54859572486944330, 1.617624508639602388 ) ) ;
#3949=CARTESIAN_POINT ( 'NONE',  ( -34.58449383169706692, -31.14859572486944828, -8.874878320068054549 ) ) ;
#3950=CARTESIAN_POINT ( 'NONE',  ( -20.12537475255788522, -36.05140427513057944, -1.507589171976365439 ) ) ;
#3953=CARTESIAN_POINT ( 'NONE',  ( -34.36011273255026310, -49.10140427513058370, 8.440510857627391061 ) ) ;
#3961=CARTESIAN_POINT ( 'NONE',  ( -28.67030704715798350, -43.80000000000000426, 8.395350895058669494 ) ) ;
#3967=CARTESIAN_POINT ( 'NONE',  ( -28.43739315969223824, -39.45000000000000995, -9.865911304835512041 ) ) ;
#3970=CARTESIAN_POINT ( 'NONE',  ( -28.54686042191934092, -35.45140427513057801, -8.818680382772479120 ) ) ;
#3974=CARTESIAN_POINT ( 'NONE',  ( -38.39535089505872634, -32.70000000000000995, -1.329692952841885267 ) ) ;
#3980=CARTESIAN_POINT ( 'NONE',  ( -38.90016716647221529, -44.85000000000001563, -4.534861676072185155 ) ) ;
#3982=CARTESIAN_POINT ( 'NONE',  ( -31.45313957808072303, -48.95140427513057091, 8.818680382772479120 ) ) ;
#3985=CARTESIAN_POINT ( 'NONE',  ( -34.26570676250101855, -39.09859572486944046, 8.488613101951703044 ) ) ;
#3993=CARTESIAN_POINT ( 'NONE',  ( -21.17260567462091458, -46.05000000000001137, -1.398121909749242331 ) ) ;
#3994=CARTESIAN_POINT ( 'NONE',  ( -31.53845232986046554, -40.29859572486944330, -9.374751783755117529 ) ) ;
#3995=CARTESIAN_POINT ( 'NONE',  ( -28.56619749409589204, -36.80140427513057944, 9.391326687552490782 ) ) ;
#3998=CARTESIAN_POINT ( 'NONE',  ( -22.89739904353894318, -44.75140427513058228, -7.023824353025938549 ) ) ;
#4006=CARTESIAN_POINT ( 'NONE',  ( -31.39812190974910422, -40.95000000000000995, 8.827394325379140483 ) ) ;
#4012=CARTESIAN_POINT ( 'NONE',  ( -38.46456197978948666, -47.40000000000001279, 4.312909747525784709 ) ) ;
#4015=CARTESIAN_POINT ( 'NONE',  ( -21.61293655684001536, -30.20140427513057446, 1.382017864820032971 ) ) ;
#4019=CARTESIAN_POINT ( 'NONE',  ( -36.01040764008574513, -33.00000000000000711, -6.010407640085605685 ) ) ;
#4026=CARTESIAN_POINT ( 'NONE',  ( -28.51387258211773812, -46.80000000000001137, 9.383039235653802379 ) ) ;
#4027=CARTESIAN_POINT ( 'NONE',  ( -38.38706344316003793, -49.70140427513058512, -1.382017864820032083 ) ) ;
#4031=CARTESIAN_POINT ( 'NONE',  ( -20.14280263777121149, -44.04859572486944330, -1.617624508639600833 ) ) ;
#4036=CARTESIAN_POINT ( 'NONE',  ( -23.68028341417693738, -45.74999999999999289, -6.319716585823198507 ) ) ;
#4038=CARTESIAN_POINT ( 'NONE',  ( -20.14280263777121149, -38.04859572486944330, -1.617624508639600833 ) ) ;
#4039=CARTESIAN_POINT ( 'NONE',  ( -25.51477047955235378, -36.65140427513058086, 8.925456012876139766 ) ) ;
#4042=CARTESIAN_POINT ( 'NONE',  ( -28.56619749409589204, -45.80140427513057944, 9.391326687552490782 ) ) ;
#4051=CARTESIAN_POINT ( 'NONE',  ( -28.65689575858256077, -34.44859572486944188, -8.836108267985801845 ) ) ;
#4052=CARTESIAN_POINT ( 'NONE',  ( -25.68709025247441602, -33.60000000000000142, -8.464561979789547053 ) ) ;
#4057=CARTESIAN_POINT ( 'NONE',  ( -20.13408869516453947, -43.04999999999999005, -1.562606840307983136 ) ) ;
#4061=CARTESIAN_POINT ( 'NONE',  ( -23.64089511245930098, -38.75140427513058228, -6.280328284105564762 ) ) ;
#4065=CARTESIAN_POINT ( 'NONE',  ( -23.98959235991431171, -43.50000000000001421, 6.010407640085604797 ) ) ;
#4070=CARTESIAN_POINT ( 'NONE',  ( -22.93678734525658314, -48.75000000000001421, -7.063212654743582952 ) ) ;
#4071=CARTESIAN_POINT ( 'NONE',  ( -24.02705286092866643, -45.50140427513058228, 6.047868141099968398 ) ) ;
#4074=CARTESIAN_POINT ( 'NONE',  ( -34.26570676250101855, -51.09859572486944046, 8.488613101951703044 ) ) ;
#4076=CARTESIAN_POINT ( 'NONE',  ( -34.53486167607238855, -33.15000000000000568, -8.900167166472096270 ) ) ;
#4079=DIRECTION ( 'NONE',  ( -0.7071067811865587860, 0.000000000000000000, -0.7071067811865362485 ) ) ;
#4080=CARTESIAN_POINT ( 'NONE',  ( -26.14108075221394856, -48.60000000000000142, -7.573555455601170827 ) ) ;
#4081=CARTESIAN_POINT ( 'NONE',  ( -39.85719736222883824, -39.54859572486944330, 1.617624508639602388 ) ) ;
#4082=CARTESIAN_POINT ( 'NONE',  ( -37.10260095646111012, -43.25140427513058228, 7.023824353025939438 ) ) ;
#4085=CARTESIAN_POINT ( 'NONE',  ( -37.10260095646111012, -43.25140427513058228, 7.023824353025939438 ) ) ;
#4094=CARTESIAN_POINT ( 'NONE',  ( -36.04786814110010340, -30.99859572486944259, -5.972947139071243861 ) ) ;
#4095=CARTESIAN_POINT ( 'NONE',  ( -34.53486167607238144, -36.15000000000001279, -8.900167166472096270 ) ) ;
#4100=CARTESIAN_POINT ( 'NONE',  ( -39.38303923565386100, -47.70000000000000284, -1.486127417882099788 ) ) ;
#4103=CARTESIAN_POINT ( 'NONE',  ( -35.97294713907137975, -44.00140427513057517, -6.047868141099968398 ) ) ;
#4104=MECHANICAL_DESIGN_GEOMETRIC_PRESENTATION_REPRESENTATION('',(#8334),#7197);
#4107=CARTESIAN_POINT ( 'NONE',  ( -28.67030704715798350, -40.80000000000000426, 8.395350895058669494 ) ) ;
#4109=CARTESIAN_POINT ( 'NONE',  ( -36.71751442127229836, -51.00000000000000711, -6.717514421272142044 ) ) ;
#4113=CARTESIAN_POINT ( 'NONE',  ( -28.51387258211773812, -49.80000000000001137, 9.383039235653802379 ) ) ;
#4114=CARTESIAN_POINT ( 'NONE',  ( -24.02705286092866643, -48.50140427513058938, 6.047868141099968398 ) ) ;
#4118=CARTESIAN_POINT ( 'NONE',  ( -39.39132668755255651, -42.69859572486944188, -1.433802505903950308 ) ) ;
#4120=CARTESIAN_POINT ( 'NONE',  ( -22.93678734525658314, -33.75000000000000711, -7.063212654743582064 ) ) ;
#4125=CARTESIAN_POINT ( 'NONE',  ( -36.01040764008574513, -51.00000000000000711, -6.010407640085605685 ) ) ;
#4126=CARTESIAN_POINT ( 'NONE',  ( -21.55948914237271907, -37.89859572486944472, -4.360112732550413206 ) ) ;
#4127=CARTESIAN_POINT ( 'NONE',  ( -39.87462524744216807, -40.55140427513058654, 1.507589171976367215 ) ) ;
#4137=EDGE_CURVE ( 'NONE', #4270, #8652, #5515, .T. ) ;
#4138=CARTESIAN_POINT ( 'NONE',  ( -28.65689575858256077, -31.44859572486944188, -8.836108267985801845 ) ) ;
#4140=CARTESIAN_POINT ( 'NONE',  ( -34.53486167607238144, -30.15000000000000213, -8.900167166472096270 ) ) ;
#4149=CARTESIAN_POINT ( 'NONE',  ( -26.09387776718931917, -44.60140427513058370, -7.549504333439021941 ) ) ;
#4152=CARTESIAN_POINT ( 'NONE',  ( -36.01040764008574513, -45.00000000000000711, -6.010407640085605685 ) ) ;
#4157=CARTESIAN_POINT ( 'NONE',  ( -20.61696076434619584, -46.20000000000000284, 1.486127417882100676 ) ) ;
#4158=CARTESIAN_POINT ( 'NONE',  ( -26.14108075221394856, -33.60000000000000142, -7.573555455601170827 ) ) ;
#4160=CARTESIAN_POINT ( 'NONE',  ( -20.14280263777121149, -50.04859572486944330, -1.617624508639600833 ) ) ;
#4162=CARTESIAN_POINT ( 'NONE',  ( -34.31290974752564438, -35.10000000000000853, 8.464561979789547053 ) ) ;
#4167=CARTESIAN_POINT ( 'NONE',  ( -21.60464910494133406, -46.20000000000000284, 1.329692952841886155 ) ) ;
#4168=CARTESIAN_POINT ( 'NONE',  ( -28.49241082802385350, -37.44859572486943478, -9.874625247442173404 ) ) ;
#4169=CARTESIAN_POINT ( 'NONE',  ( -34.36011273255026310, -40.10140427513057659, 8.440510857627391061 ) ) ;
#4171=EDGE_LOOP ( 'NONE', ( #4491, #5726 ) ) ;
#4179=CARTESIAN_POINT ( 'NONE',  ( -23.98959235991431171, -49.50000000000000711, 6.010407640085604797 ) ) ;
#4180=CARTESIAN_POINT ( 'NONE',  ( -39.86591130483550671, -35.55000000000001137, 1.562606840307984468 ) ) ;
#4183=CARTESIAN_POINT ( 'NONE',  ( -31.56260684030781505, -49.95000000000000995, 9.865911304835510265 ) ) ;
#4190=CARTESIAN_POINT ( 'NONE',  ( -31.27736804086391942, -41.30140427513058654, -8.403638346957361449 ) ) ;
#4193=CARTESIAN_POINT ( 'NONE',  ( -33.85891924778610473, -47.10000000000000142, 7.573555455601171715 ) ) ;
#4200=CARTESIAN_POINT ( 'NONE',  ( -23.98959235991431171, -40.50000000000000711, 6.010407640085604797 ) ) ;
#4203=CARTESIAN_POINT ( 'NONE',  ( -34.26570676250101855, -48.09859572486944046, 8.488613101951703044 ) ) ;
#4209=CARTESIAN_POINT ( 'NONE',  ( -28.65689575858256077, -43.44859572486944188, -8.836108267985801845 ) ) ;
#4210=CARTESIAN_POINT ( 'NONE',  ( -39.85719736222883824, -48.54859572486944330, 1.617624508639602388 ) ) ;
#4211=CARTESIAN_POINT ( 'NONE',  ( -39.87462524744216807, -49.55140427513056522, 1.507589171976367215 ) ) ;
#4221=CARTESIAN_POINT ( 'NONE',  ( -22.45049566656107842, -31.89859572486943762, -3.906122232810846917 ) ) ;
#4222=CARTESIAN_POINT ( 'NONE',  ( -25.68709025247441602, -36.60000000000000853, -8.464561979789547053 ) ) ;
#4224=CARTESIAN_POINT ( 'NONE',  ( -39.38303923565386100, -47.70000000000000284, -1.486127417882099788 ) ) ;
#4232=CARTESIAN_POINT ( 'NONE',  ( -36.35910488754074521, -46.25140427513058228, 6.280328284105565650 ) ) ;
#4238=CARTESIAN_POINT ( 'NONE',  ( -21.60464910494133406, -49.20000000000000995, 1.329692952841886155 ) ) ;
#4242=CARTESIAN_POINT ( 'NONE',  ( -21.17260567462091458, -34.04999999999998295, -1.398121909749242331 ) ) ;
#4246=CARTESIAN_POINT ( 'NONE',  ( -22.93678734525658314, -33.75000000000001421, -7.063212654743582952 ) ) ;
#4254=CARTESIAN_POINT ( 'NONE',  ( -22.01140368885771892, -35.34859572486944046, 4.007875659808335378 ) ) ;
#4255=CARTESIAN_POINT ( 'NONE',  ( -25.73429323749904185, -49.59859572486944046, -8.488613101951701267 ) ) ;
#4256=CARTESIAN_POINT ( 'NONE',  ( -28.72263195913613387, -33.80140427513056522, 8.403638346957361449 ) ) ;
#4257=ADVANCED_FACE ( 'NONE', ( #5839 ), #1038, .T. ) ;
#4266=CARTESIAN_POINT ( 'NONE',  ( -33.81171626276147890, -42.09859572486944046, 7.597606577763319713 ) ) ;
#4267=CARTESIAN_POINT ( 'NONE',  ( -36.71751442127229836, -42.00000000000000711, -6.717514421272142044 ) ) ;
#4270=VERTEX_POINT ( 'NONE', #369 ) ;
#4271=CARTESIAN_POINT ( 'NONE',  ( -31.56260684030781505, -43.95000000000000284, 9.865911304835510265 ) ) ;
#4278=CARTESIAN_POINT ( 'NONE',  ( -22.03669253526174998, -31.34999999999999787, 4.057507815433014642 ) ) ;
#4285=CARTESIAN_POINT ( 'NONE',  ( -22.03669253526174998, -34.35000000000000853, 4.057507815433014642 ) ) ;
#4288=CARTESIAN_POINT ( 'NONE',  ( -34.31290974752564438, -35.10000000000000853, 8.464561979789547053 ) ) ;
#4291=CARTESIAN_POINT ( 'NONE',  ( -22.93678734525658314, -36.75000000000000711, -7.063212654743582064 ) ) ;
#4295=CARTESIAN_POINT ( 'NONE',  ( -26.18828373723858149, -34.59859572486944046, -7.597606577763319713 ) ) ;
#4296=CARTESIAN_POINT ( 'NONE',  ( -25.41550616830297571, -47.64859572486945183, 8.874878320068054549 ) ) ;
#4297=CARTESIAN_POINT ( 'NONE',  ( -37.10260095646111012, -49.25140427513058938, 7.023824353025939438 ) ) ;
#4309=CARTESIAN_POINT ( 'NONE',  ( -31.38201786482021305, -37.29859572486943620, -8.387063443159975762 ) ) ;
#4310=CARTESIAN_POINT ( 'NONE',  ( -28.51387258211773812, -46.80000000000001137, 9.383039235653802379 ) ) ;
#4313=CARTESIAN_POINT ( 'NONE',  ( -28.43739315969223824, -45.45000000000000995, -9.865911304835512041 ) ) ;
#4322=CARTESIAN_POINT ( 'NONE',  ( -31.32969295284206979, -33.30000000000000426, -8.395350895058669494 ) ) ;
#4333=CARTESIAN_POINT ( 'NONE',  ( -37.96330746473829976, -41.84999999999999432, -4.057507815433013754 ) ) ;
#4336=CARTESIAN_POINT ( 'NONE',  ( -23.28248557872775137, -34.50000000000000000, 6.717514421272141156 ) ) ;
#4338=CARTESIAN_POINT ( 'NONE',  ( -31.48612741788231517, -45.30000000000000426, -9.383039235653804155 ) ) ;
#4343=CARTESIAN_POINT ( 'NONE',  ( -36.04786814110010340, -36.99859572486943193, -5.972947139071243861 ) ) ;
#4344=CARTESIAN_POINT ( 'NONE',  ( -31.53845232986046554, -46.29859572486944330, -9.374751783755117529 ) ) ;
#4345=CARTESIAN_POINT ( 'NONE',  ( -39.37475178375516549, -46.70140427513057801, -1.538452329860249712 ) ) ;
#4356=CARTESIAN_POINT ( 'NONE',  ( -23.71967171589458445, -43.74859572486943904, -6.359104887540838469 ) ) ;
#4357=CARTESIAN_POINT ( 'NONE',  ( -34.31290974752564438, -47.10000000000000142, 8.464561979789547053 ) ) ;
#4359=CARTESIAN_POINT ( 'NONE',  ( -28.51387258211773812, -43.80000000000000426, 9.383039235653802379 ) ) ;
#4366=CARTESIAN_POINT ( 'NONE',  ( -37.57355545560112375, -32.40000000000000568, 3.858919247786223305 ) ) ;
#4374=CARTESIAN_POINT ( 'NONE',  ( -25.94249218456686279, -40.65000000000000568, 7.963307464738195840 ) ) ;
#4379=CARTESIAN_POINT ( 'NONE',  ( -20.61696076434619584, -37.20000000000000284, 1.486127417882100676 ) ) ;
#4382=CARTESIAN_POINT ( 'NONE',  ( -34.53486167607238855, -42.15000000000000568, -8.900167166472096270 ) ) ;
#4386=CARTESIAN_POINT ( 'NONE',  ( -21.59636165304264921, -47.19859572486943478, 1.277368040863740228 ) ) ;
#4387=CARTESIAN_POINT ( 'NONE',  ( -28.43739315969223824, -30.44999999999999574, -9.865911304835512041 ) ) ;
#4388=CARTESIAN_POINT ( 'NONE',  ( -37.59760657776328685, -34.40140427513058086, 3.811716262761598362 ) ) ;
#4391=CARTESIAN_POINT ( 'NONE',  ( -21.09983283352784156, -34.35000000000000853, 4.534861676072186043 ) ) ;
#4397=CARTESIAN_POINT ( 'NONE',  ( -21.18131961722757595, -41.04859572486944330, -1.453139578080854699 ) ) ;
#4398=CARTESIAN_POINT ( 'NONE',  ( -39.38303923565386100, -47.70000000000000284, -1.486127417882099788 ) ) ;
#4401=CARTESIAN_POINT ( 'NONE',  ( -28.38237549136062654, -32.45140427513058512, -9.857197362228843573 ) ) ;
#4409=CARTESIAN_POINT ( 'NONE',  ( -21.17260567462091458, -37.05000000000001137, -1.398121909749242331 ) ) ;
#4419=CARTESIAN_POINT ( 'NONE',  ( -23.98959235991431171, -43.50000000000001421, 6.010407640085604797 ) ) ;
#4423=CARTESIAN_POINT ( 'NONE',  ( -38.90016716647221529, -38.85000000000001563, -4.534861676072185155 ) ) ;
#4426=CARTESIAN_POINT ( 'NONE',  ( -25.68709025247441602, -42.60000000000000853, -8.464561979789547053 ) ) ;
#4429=CARTESIAN_POINT ( 'NONE',  ( -38.40363834695740053, -51.69859572486944188, -1.277368040863739118 ) ) ;
#4430=CARTESIAN_POINT ( 'NONE',  ( -31.48612741788231517, -39.30000000000001137, -9.383039235653804155 ) ) ;
#4431=CARTESIAN_POINT ( 'NONE',  ( -31.27736804086391942, -35.30140427513057944, -8.403638346957361449 ) ) ;
#4434=CARTESIAN_POINT ( 'NONE',  ( -31.48612741788231517, -33.30000000000000426, -9.383039235653804155 ) ) ;
#4441=CARTESIAN_POINT ( 'NONE',  ( -37.98859631114233792, -36.84859572486944046, -4.007875659808334490 ) ) ;
#4442=CARTESIAN_POINT ( 'NONE',  ( -28.43739315969223824, -42.44999999999999574, -9.865911304835512041 ) ) ;
#4444=CARTESIAN_POINT ( 'NONE',  ( -34.36011273255026310, -31.10140427513058370, 8.440510857627391061 ) ) ;
#4451=CARTESIAN_POINT ( 'NONE',  ( -28.72263195913613387, -48.80140427513057233, 8.403638346957361449 ) ) ;
#4463=CARTESIAN_POINT ( 'NONE',  ( -31.48612741788231517, -42.30000000000000426, -9.383039235653804155 ) ) ;
#4467=CARTESIAN_POINT ( 'NONE',  ( -20.60867331244750034, -32.19859572486942767, 1.433802505903951419 ) ) ;
#4468=CARTESIAN_POINT ( 'NONE',  ( -38.90016716647221529, -38.85000000000001563, -4.534861676072185155 ) ) ;
#4469=CARTESIAN_POINT ( 'NONE',  ( -31.45313957808072303, -42.95140427513058512, 8.818680382772479120 ) ) ;
#4473=CARTESIAN_POINT ( 'NONE',  ( -39.86591130483550671, -38.54999999999999716, 1.562606840307984468 ) ) ;
#4480=CARTESIAN_POINT ( 'NONE',  ( -21.18131961722757595, -47.04859572486944330, -1.453139578080854699 ) ) ;
#4481=CARTESIAN_POINT ( 'NONE',  ( -34.48522952044771017, -29.15140427513058441, -8.925456012876139766 ) ) ;
#4483=CARTESIAN_POINT ( 'NONE',  ( -38.48861310195163554, -34.40140427513058086, 4.265706762501153548 ) ) ;
#4491=ORIENTED_EDGE ( 'NONE', *, *, #4736, .F. ) ;
#4492=CARTESIAN_POINT ( 'NONE',  ( -26.14108075221394856, -42.60000000000000853, -7.573555455601170827 ) ) ;
#4501=CARTESIAN_POINT ( 'NONE',  ( -22.03669253526174998, -40.34999999999999432, 4.057507815433014642 ) ) ;
#4507=CARTESIAN_POINT ( 'NONE',  ( -23.71967171589458445, -49.74859572486944614, -6.359104887540838469 ) ) ;
#4508=CARTESIAN_POINT ( 'NONE',  ( -21.53543802021056663, -33.90000000000000568, -4.312909747525783821 ) ) ;
#4509=CARTESIAN_POINT ( 'NONE',  ( -38.38706344316003793, -43.70140427513058512, -1.382017864820032083 ) ) ;
#4513=CARTESIAN_POINT ( 'NONE',  ( -25.41550616830297571, -35.64859572486943051, 8.874878320068054549 ) ) ;
#4514=CARTESIAN_POINT ( 'NONE',  ( -25.68709025247441602, -39.60000000000000853, -8.464561979789547053 ) ) ;
#4522=CARTESIAN_POINT ( 'NONE',  ( -28.61798213517984024, -47.79859572486944330, 8.387063443159973986 ) ) ;
#4523=CARTESIAN_POINT ( 'NONE',  ( -25.63988726744978663, -32.60140427513057659, -8.440510857627391061 ) ) ;
#4527=CARTESIAN_POINT ( 'NONE',  ( -20.12537475255788522, -33.05140427513057233, -1.507589171976365439 ) ) ;
#4536=CARTESIAN_POINT ( 'NONE',  ( -21.17260567462091458, -40.05000000000001137, -1.398121909749242331 ) ) ;
#4541=CARTESIAN_POINT ( 'NONE',  ( -28.72263195913613387, -36.80140427513057944, 8.403638346957361449 ) ) ;
#4545=CARTESIAN_POINT ( 'NONE',  ( -22.42644454439892598, -33.90000000000000568, -3.858919247786222861 ) ) ;
#4552=CARTESIAN_POINT ( 'NONE',  ( -34.10713997105786888, -49.14859572486945183, -7.938018618334151455 ) ) ;
#4553=CARTESIAN_POINT ( 'NONE',  ( -31.56260684030781505, -31.95000000000000639, 9.865911304835510265 ) ) ;
#4554=CARTESIAN_POINT ( 'NONE',  ( -21.61293655684001536, -42.20140427513058512, 1.382017864820032971 ) ) ;
#4559=CARTESIAN_POINT ( 'NONE',  ( -23.24502507771338600, -38.49859572486943904, 6.680053920257780220 ) ) ;
#4560=CARTESIAN_POINT ( 'NONE',  ( -37.06321265474346660, -38.25000000000001421, 7.063212654743582952 ) ) ;
#4567=CARTESIAN_POINT ( 'NONE',  ( -28.49241082802385350, -31.44859572486944188, -9.874625247442173404 ) ) ;
#4568=CARTESIAN_POINT ( 'NONE',  ( -28.38237549136062654, -29.45140427513057801, -9.857197362228843573 ) ) ;
#4572=CARTESIAN_POINT ( 'NONE',  ( -31.43380250590416125, -32.30140427513056522, -9.391326687552492558 ) ) ;
#4576=CARTESIAN_POINT ( 'NONE',  ( -36.36396103067902175, -30.00000000000000711, -6.363961030678874309 ) ) ;
#4580=CARTESIAN_POINT ( 'NONE',  ( -38.39535089505872634, -38.70000000000000284, -1.329692952841885267 ) ) ;
#4583=CARTESIAN_POINT ( 'NONE',  ( -34.53486167607238144, -48.15000000000001279, -8.900167166472096270 ) ) ;
#4587=CARTESIAN_POINT ( 'NONE',  ( -31.27736804086391942, -35.30140427513057944, -8.403638346957361449 ) ) ;
#4590=CARTESIAN_POINT ( 'NONE',  ( -23.68028341417693738, -33.75000000000000711, -6.319716585823200283 ) ) ;
#4593=CARTESIAN_POINT ( 'NONE',  ( -37.06321265474346660, -50.24999999999999289, 7.063212654743582952 ) ) ;
#4597=CARTESIAN_POINT ( 'NONE',  ( -23.28248557872775137, -34.50000000000000000, 6.717514421272141156 ) ) ;
#4598=CARTESIAN_POINT ( 'NONE',  ( -28.72263195913613387, -39.80140427513057944, 8.403638346957361449 ) ) ;
#4602=CARTESIAN_POINT ( 'NONE',  ( -28.49241082802385350, -34.44859572486944188, -9.874625247442173404 ) ) ;
#4603=CARTESIAN_POINT ( 'NONE',  ( -22.93678734525658314, -42.75000000000001421, -7.063212654743582952 ) ) ;
#4609=CARTESIAN_POINT ( 'NONE',  ( -38.40363834695740053, -51.69859572486944188, -1.277368040863739118 ) ) ;
#4610=CARTESIAN_POINT ( 'NONE',  ( -31.61762450863942320, -33.95140427513058512, 9.857197362228843573 ) ) ;
#4614=CARTESIAN_POINT ( 'NONE',  ( -25.63988726744978663, -44.60140427513058370, -8.440510857627391061 ) ) ;
#4621=CARTESIAN_POINT ( 'NONE',  ( -38.39535089505872634, -41.70000000000000995, -1.329692952841885267 ) ) ;
#4626=CARTESIAN_POINT ( 'NONE',  ( -28.51387258211773812, -46.80000000000001137, 9.383039235653802379 ) ) ;
#4629=CARTESIAN_POINT ( 'NONE',  ( -22.40239342223677355, -29.90140427513058796, -3.811716262761597473 ) ) ;
#4631=CARTESIAN_POINT ( 'NONE',  ( -22.42644454439892598, -36.90000000000000568, -3.858919247786222861 ) ) ;
#4637=CARTESIAN_POINT ( 'NONE',  ( -21.09983283352784156, -43.35000000000000853, 4.534861676072186043 ) ) ;
#4638=CARTESIAN_POINT ( 'NONE',  ( -33.90612223281073057, -46.10140427513058370, 7.549504333439023718 ) ) ;
#4642=CARTESIAN_POINT ( 'NONE',  ( -21.55948914237271907, -37.89859572486944472, -4.360112732550413206 ) ) ;
#4650=CARTESIAN_POINT ( 'NONE',  ( -38.81868038277247734, -33.54859572486944330, 1.453139578080855365 ) ) ;
#4651=CARTESIAN_POINT ( 'NONE',  ( -21.55948914237271907, -31.89859572486943762, -4.360112732550413206 ) ) ;
#4652=CARTESIAN_POINT ( 'NONE',  ( -23.31994607974211675, -39.50140427513058228, 6.754974922286503869 ) ) ;
#4656=CARTESIAN_POINT ( 'NONE',  ( -20.62524821624488069, -48.20140427513058512, 1.538452329860250378 ) ) ;
#4663=CARTESIAN_POINT ( 'NONE',  ( -28.60187809025093841, -39.45000000000000995, -8.827394325379140483 ) ) ;
#4670=CARTESIAN_POINT ( 'NONE',  ( -22.93678734525658314, -48.75000000000001421, -7.063212654743582952 ) ) ;
#4673=CARTESIAN_POINT ( 'NONE',  ( -22.06198138166579170, -30.35140427513058015, 4.107139971057695682 ) ) ;
#4678=CARTESIAN_POINT ( 'NONE',  ( -28.67030704715798350, -31.80000000000000782, 8.395350895058669494 ) ) ;
#4686=CARTESIAN_POINT ( 'NONE',  ( -34.53486167607238144, -45.14999999999999858, -8.900167166472096270 ) ) ;
#4687=CARTESIAN_POINT ( 'NONE',  ( -22.40239342223677355, -47.90140427513058086, -3.811716262761597473 ) ) ;
#4692=CARTESIAN_POINT ( 'NONE',  ( -28.49241082802385350, -49.44859572486943478, -9.874625247442173404 ) ) ;
#4699=CARTESIAN_POINT ( 'NONE',  ( -36.04786814110010340, -33.99859572486943904, -5.972947139071243861 ) ) ;
#4700=CARTESIAN_POINT ( 'NONE',  ( -38.44051085762733777, -42.39859572486944472, 4.360112732550414982 ) ) ;
#4701=CARTESIAN_POINT ( 'NONE',  ( -36.68005392025794009, -44.00140427513057517, -6.754974922286504757 ) ) ;
#4704=CARTESIAN_POINT ( 'NONE',  ( -23.31994607974211675, -45.50140427513058228, 6.754974922286503869 ) ) ;
#4713=CARTESIAN_POINT ( 'NONE',  ( -28.67030704715798350, -49.80000000000001137, 8.395350895058669494 ) ) ;
#4714=CARTESIAN_POINT ( 'NONE',  ( -21.09983283352784156, -37.35000000000000853, 4.534861676072186043 ) ) ;
#4718=CARTESIAN_POINT ( 'NONE',  ( -34.31290974752564438, -41.10000000000000142, 8.464561979789547053 ) ) ;
#4720=CARTESIAN_POINT ( 'NONE',  ( -28.54686042191934092, -32.45140427513058512, -8.818680382772479120 ) ) ;
#4724=CARTESIAN_POINT ( 'NONE',  ( -22.42644454439892598, -42.90000000000000568, -3.858919247786222861 ) ) ;
#4730=CARTESIAN_POINT ( 'NONE',  ( -21.09983283352784156, -46.34999999999998721, 4.534861676072186043 ) ) ;
#4731=CARTESIAN_POINT ( 'NONE',  ( -38.38706344316003793, -46.70140427513057801, -1.382017864820032083 ) ) ;
#4735=CARTESIAN_POINT ( 'NONE',  ( -20.60867331244750034, -50.19859572486944188, 1.433802505903951419 ) ) ;
#4736=EDGE_CURVE ( 'NONE', #7915, #8652, #416, .T. ) ;
#4738=CARTESIAN_POINT ( 'NONE',  ( -39.86591130483550671, -32.55000000000000426, 1.562606840307984690 ) ) ;
#4741=CARTESIAN_POINT ( 'NONE',  ( -26.14108075221394856, -45.60000000000000853, -7.573555455601170827 ) ) ;
#4742=CARTESIAN_POINT ( 'NONE',  ( -25.41550616830297571, -35.64859572486943051, 8.874878320068054549 ) ) ;
#4743=CARTESIAN_POINT ( 'NONE',  ( -23.31994607974211675, -45.50140427513058228, 6.754974922286503869 ) ) ;
#4746=CARTESIAN_POINT ( 'NONE',  ( -28.38237549136062654, -41.45140427513058512, -9.857197362228843573 ) ) ;
#4755=CARTESIAN_POINT ( 'NONE',  ( -34.10713997105786888, -34.14859572486943051, -7.938018618334151455 ) ) ;
#4756=CARTESIAN_POINT ( 'NONE',  ( -38.46456197978948666, -38.40000000000000568, 4.312909747525784709 ) ) ;
#4762=CARTESIAN_POINT ( 'NONE',  ( -31.48612741788231517, -45.30000000000000426, -9.383039235653804155 ) ) ;
#4766=CARTESIAN_POINT ( 'NONE',  ( -31.27736804086391942, -44.30140427513057944, -8.403638346957361449 ) ) ;
#4768=CARTESIAN_POINT ( 'NONE',  ( -34.05750781543319050, -45.15000000000000568, -7.963307464738194952 ) ) ;
#4774=CARTESIAN_POINT ( 'NONE',  ( -39.38303923565386100, -47.70000000000000284, -1.486127417882099788 ) ) ;
#4775=CARTESIAN_POINT ( 'NONE',  ( -37.96330746473829976, -32.85000000000000853, -4.057507815433013754 ) ) ;
#4778=CARTESIAN_POINT ( 'NONE',  ( -39.39132668755255651, -48.69859572486944188, -1.433802505903950308 ) ) ;
#4780=CARTESIAN_POINT ( 'NONE',  ( -36.36396103067902175, -51.00000000000000711, -6.363961030678874309 ) ) ;
#4781=CARTESIAN_POINT ( 'NONE',  ( -38.46456197978948666, -32.40000000000000568, 4.312909747525784709 ) ) ;
#4785=CARTESIAN_POINT ( 'NONE',  ( -37.57355545560112375, -47.40000000000001279, 3.858919247786223305 ) ) ;
#4786=CARTESIAN_POINT ( 'NONE',  ( -37.02382435302582309, -42.24859572486943904, 7.102600956461226467 ) ) ;
#4787=CARTESIAN_POINT ( 'NONE',  ( -20.12537475255788522, -42.05140427513057944, -1.507589171976365439 ) ) ;
#4799=CARTESIAN_POINT ( 'NONE',  ( -37.57355545560112375, -50.40000000000000568, 3.858919247786223305 ) ) ;
#4800=CARTESIAN_POINT ( 'NONE',  ( -34.53486167607238144, -39.14999999999999147, -8.900167166472096270 ) ) ;
#4806=CARTESIAN_POINT ( 'NONE',  ( -34.31290974752564438, -50.10000000000000853, 8.464561979789547053 ) ) ;
#4809=CARTESIAN_POINT ( 'NONE',  ( -37.59760657776328685, -43.40140427513058796, 3.811716262761598362 ) ) ;
#4812=CARTESIAN_POINT ( 'NONE',  ( -38.39535089505872634, -41.70000000000000995, -1.329692952841885267 ) ) ;
#4817=CARTESIAN_POINT ( 'NONE',  ( -25.46513832392765408, -49.64999999999999147, 8.900167166472096270 ) ) ;
#4819=CARTESIAN_POINT ( 'NONE',  ( -25.99212434019154472, -45.65140427513058086, 7.988596311142242890 ) ) ;
#4824=CARTESIAN_POINT ( 'NONE',  ( -25.73429323749904185, -49.59859572486944046, -8.488613101951701267 ) ) ;
#4826=CARTESIAN_POINT ( 'NONE',  ( -36.71751442127229836, -30.00000000000000711, -6.717514421272142044 ) ) ;
#4828=AXIS2_PLACEMENT_3D ( 'NONE', #2817, #6248, #8154 ) ;
#4833=CARTESIAN_POINT ( 'NONE',  ( -37.96330746473829976, -50.84999999999999432, -4.057507815433013754 ) ) ;
#4834=CARTESIAN_POINT ( 'NONE',  ( -34.26570676250101855, -42.09859572486944046, 8.488613101951703044 ) ) ;
#4835=CARTESIAN_POINT ( 'NONE',  ( -28.38237549136062654, -41.45140427513058512, -9.857197362228843573 ) ) ;
#4846=CARTESIAN_POINT ( 'NONE',  ( -31.34310424141748896, -35.94859572486944188, 8.836108267985801845 ) ) ;
#4847=CARTESIAN_POINT ( 'NONE',  ( -34.31290974752564438, -35.10000000000000853, 8.464561979789547053 ) ) ;
#4850=CARTESIAN_POINT ( 'NONE',  ( -22.93678734525658314, -48.75000000000001421, -7.063212654743582952 ) ) ;
#4857=CARTESIAN_POINT ( 'NONE',  ( -21.16389173201424612, -42.05140427513057944, -1.343104241417630185 ) ) ;
#4861=CARTESIAN_POINT ( 'NONE',  ( -38.82739432537914581, -41.55000000000000426, 1.398121909749243663 ) ) ;
#4865=SURFACE_STYLE_FILL_AREA ( #6308 ) ;
#4867=CARTESIAN_POINT ( 'NONE',  ( -28.60187809025093841, -39.45000000000000995, -8.827394325379140483 ) ) ;
#4871=CARTESIAN_POINT ( 'NONE',  ( -39.39132668755255651, -51.69859572486944188, -1.433802505903950308 ) ) ;
#4873=CARTESIAN_POINT ( 'NONE',  ( -37.06321265474346660, -32.25000000000000711, 7.063212654743582952 ) ) ;
#4876=CARTESIAN_POINT ( 'NONE',  ( -21.59636165304264921, -41.19859572486944188, 1.277368040863740228 ) ) ;
#4877=CARTESIAN_POINT ( 'NONE',  ( -25.73429323749904185, -37.59859572486943335, -8.488613101951701267 ) ) ;
#4878=CARTESIAN_POINT ( 'NONE',  ( -38.83610826798580717, -34.55140427513057233, 1.343104241417631073 ) ) ;
#4881=CARTESIAN_POINT ( 'NONE',  ( -28.43739315969223824, -30.44999999999999574, -9.865911304835512041 ) ) ;
#4889=CARTESIAN_POINT ( 'NONE',  ( -36.28032828410546529, -33.24859572486943193, 6.359104887540839357 ) ) ;
#4890=CARTESIAN_POINT ( 'NONE',  ( -31.56260684030781505, -31.95000000000000639, 9.865911304835510265 ) ) ;
#4892=CARTESIAN_POINT ( 'NONE',  ( -23.28248557872775137, -49.50000000000000711, 6.717514421272141156 ) ) ;
#4896=STYLED_ITEM ( 'NONE', ( #2267 ), #5903 ) ;
#4899=CARTESIAN_POINT ( 'NONE',  ( -22.40239342223677355, -44.90140427513058086, -3.811716262761597473 ) ) ;
#4903=CARTESIAN_POINT ( 'NONE',  ( -31.39812190974910422, -40.95000000000000995, 8.827394325379140483 ) ) ;
#4905=CARTESIAN_POINT ( 'NONE',  ( -26.14108075221394856, -39.60000000000000853, -7.573555455601170827 ) ) ;
#4909=CARTESIAN_POINT ( 'NONE',  ( -23.28248557872775137, -31.50000000000000711, 6.717514421272141156 ) ) ;
#4911=CARTESIAN_POINT ( 'NONE',  ( -38.90016716647221529, -35.85000000000000142, -4.534861676072185155 ) ) ;
#4916=CARTESIAN_POINT ( 'NONE',  ( -37.54950433343896776, -39.39859572486943762, 3.906122232810848249 ) ) ;
#4917=CARTESIAN_POINT ( 'NONE',  ( -25.41550616830297571, -50.64859572486944472, 8.874878320068054549 ) ) ;
#4918=CARTESIAN_POINT ( 'NONE',  ( -28.38237549136062654, -47.45140427513057091, -9.857197362228843573 ) ) ;
#4921=CARTESIAN_POINT ( 'NONE',  ( -21.53543802021056663, -30.90000000000000924, -4.312909747525783821 ) ) ;
#4927=CARTESIAN_POINT ( 'NONE',  ( -25.89286002894218086, -38.64859572486943762, 7.938018618334153231 ) ) ;
#4928=CARTESIAN_POINT ( 'NONE',  ( -39.86591130483550671, -41.55000000000001137, 1.562606840307984468 ) ) ;
#4930=CARTESIAN_POINT ( 'NONE',  ( -39.38303923565386100, -50.70000000000000995, -1.486127417882099788 ) ) ;
#4938=CARTESIAN_POINT ( 'NONE',  ( -36.31971658582311591, -32.25000000000000711, 6.319716585823199395 ) ) ;
#4948=CARTESIAN_POINT ( 'NONE',  ( -21.60464910494133406, -43.20000000000000995, 1.329692952841886155 ) ) ;
#4951=CARTESIAN_POINT ( 'NONE',  ( -22.93678734525658314, -42.75000000000001421, -7.063212654743582952 ) ) ;
#4953=CARTESIAN_POINT ( 'NONE',  ( -20.13408869516453947, -34.04999999999998295, -1.562606840307983136 ) ) ;
#4955=CARTESIAN_POINT ( 'NONE',  ( -21.09983283352783801, -40.34999999999999432, 4.534861676072186043 ) ) ;
#4959=CARTESIAN_POINT ( 'NONE',  ( -38.81868038277247734, -42.54859572486944330, 1.453139578080855365 ) ) ;
#4961=CARTESIAN_POINT ( 'NONE',  ( -39.39132668755255651, -48.69859572486944188, -1.433802505903950308 ) ) ;
#4962=CARTESIAN_POINT ( 'NONE',  ( -21.61293655684001536, -33.20140427513057091, 1.382017864820032971 ) ) ;
#4964=CARTESIAN_POINT ( 'NONE',  ( -22.93678734525658314, -30.75000000000000000, -7.063212654743582952 ) ) ;
#4972=CARTESIAN_POINT ( 'NONE',  ( -21.59636165304264921, -44.19859572486944899, 1.277368040863740228 ) ) ;
#4974=CARTESIAN_POINT ( 'NONE',  ( -20.61696076434619584, -46.20000000000000284, 1.486127417882100676 ) ) ;
#4978=CARTESIAN_POINT ( 'NONE',  ( -21.51138689804841420, -29.90140427513058796, -4.265706762501151772 ) ) ;
#4985=CARTESIAN_POINT ( 'NONE',  ( -36.01040764008574513, -30.00000000000000711, -6.010407640085605685 ) ) ;
#4989=CARTESIAN_POINT ( 'NONE',  ( -38.39535089505872634, -50.70000000000000995, -1.329692952841885267 ) ) ;
#4992=CARTESIAN_POINT ( 'NONE',  ( -38.39535089505872634, -38.70000000000000284, -1.329692952841885267 ) ) ;
#4996=CARTESIAN_POINT ( 'NONE',  ( -28.51387258211773812, -31.80000000000000782, 9.383039235653802379 ) ) ;
#4998=CARTESIAN_POINT ( 'NONE',  ( -39.38303923565386100, -44.70000000000000284, -1.486127417882099788 ) ) ;
#5002=CARTESIAN_POINT ( 'NONE',  ( -37.54950433343896776, -42.39859572486944472, 3.906122232810848249 ) ) ;
#5003=CARTESIAN_POINT ( 'NONE',  ( -20.60867331244750034, -47.19859572486943478, 1.433802505903951419 ) ) ;
#5004=CARTESIAN_POINT ( 'NONE',  ( -31.27736804086391942, -32.30140427513056522, -8.403638346957361449 ) ) ;
#5016=CARTESIAN_POINT ( 'NONE',  ( -34.10713997105786888, -40.14859572486943762, -7.938018618334151455 ) ) ;
#5017=CARTESIAN_POINT ( 'NONE',  ( -28.43739315969223824, -45.45000000000000995, -9.865911304835512041 ) ) ;
#5019=CARTESIAN_POINT ( 'NONE',  ( -28.56619749409589204, -30.80140427513057233, 9.391326687552490782 ) ) ;
#5027=CARTESIAN_POINT ( 'NONE',  ( -23.98959235991431171, -31.50000000000000711, 6.010407640085604797 ) ) ;
#5035=CARTESIAN_POINT ( 'NONE',  ( -28.60187809025093841, -36.45000000000000284, -8.827394325379140483 ) ) ;
#5038=CARTESIAN_POINT ( 'NONE',  ( -21.09983283352784156, -31.34999999999999787, 4.534861676072186043 ) ) ;
#5040=CARTESIAN_POINT ( 'NONE',  ( -38.46456197978948666, -41.40000000000000568, 4.312909747525784709 ) ) ;
#5041=FILL_AREA_STYLE_COLOUR ( '', #3405 ) ;
#5043=ORIENTED_EDGE ( 'NONE', *, *, #7792, .T. ) ;
#5044=CARTESIAN_POINT ( 'NONE',  ( -36.28032828410546529, -39.24859572486943904, 6.359104887540839357 ) ) ;
#5045=CARTESIAN_POINT ( 'NONE',  ( -23.24502507771338600, -44.49859572486944614, 6.680053920257780220 ) ) ;
#5046=CARTESIAN_POINT ( 'NONE',  ( -36.35910488754074521, -34.25140427513057517, 6.280328284105565650 ) ) ;
#5050=CARTESIAN_POINT ( 'NONE',  ( -28.51387258211773812, -40.80000000000000426, 9.383039235653802379 ) ) ;
#5056=CARTESIAN_POINT ( 'NONE',  ( -36.04786814110010340, -39.99859572486943904, -5.972947139071243861 ) ) ;
#5057=CARTESIAN_POINT ( 'NONE',  ( -38.90016716647221529, -47.85000000000000853, -4.534861676072185155 ) ) ;
#5059=CARTESIAN_POINT ( 'NONE',  ( -31.61762450863942320, -39.95140427513058512, 9.857197362228843573 ) ) ;
#5068=CARTESIAN_POINT ( 'NONE',  ( -37.96330746473829976, -32.85000000000000853, -4.057507815433013754 ) ) ;
#5075=CARTESIAN_POINT ( 'NONE',  ( -38.39535089505872634, -44.70000000000000284, -1.329692952841885267 ) ) ;
#5076=PRODUCT_DEFINITION_SHAPE ( 'NONE', 'NONE',  #6796 ) ;
#5079=CARTESIAN_POINT ( 'NONE',  ( -28.60187809025093841, -30.44999999999999574, -8.827394325379140483 ) ) ;
#5080=CARTESIAN_POINT ( 'NONE',  ( -20.13408869516453947, -37.05000000000001137, -1.562606840307983136 ) ) ;
#5083=CARTESIAN_POINT ( 'NONE',  ( -31.48612741788231517, -39.30000000000001137, -9.383039235653804155 ) ) ;
#5086=CARTESIAN_POINT ( 'NONE',  ( -23.71967171589458445, -46.74859572486943904, -6.359104887540838469 ) ) ;
#5087=CARTESIAN_POINT ( 'NONE',  ( -20.61696076434619584, -37.20000000000000284, 1.486127417882100676 ) ) ;
#5088=CARTESIAN_POINT ( 'NONE',  ( -28.54686042191934092, -38.45140427513057801, -8.818680382772479120 ) ) ;
#5092=CARTESIAN_POINT ( 'NONE',  ( -38.46456197978948666, -41.40000000000000568, 4.312909747525784709 ) ) ;
#5100=CARTESIAN_POINT ( 'NONE',  ( -37.98859631114233792, -45.84859572486944046, -4.007875659808334490 ) ) ;
#5101=CARTESIAN_POINT ( 'NONE',  ( -20.13408869516453947, -49.04999999999999716, -1.562606840307983136 ) ) ;
#5104=CARTESIAN_POINT ( 'NONE',  ( -28.38237549136062654, -38.45140427513057801, -9.857197362228843573 ) ) ;
#5110=CARTESIAN_POINT ( 'NONE',  ( -37.93801861833426159, -49.85140427513058370, -4.107139971057695682 ) ) ;
#5126=CARTESIAN_POINT ( 'NONE',  ( -25.68709025247441602, -39.60000000000000853, -8.464561979789547053 ) ) ;
#5129=CARTESIAN_POINT ( 'NONE',  ( -31.38201786482021305, -49.29859572486945041, -8.387063443159975762 ) ) ;
#5130=CARTESIAN_POINT ( 'NONE',  ( -39.86591130483550671, -35.55000000000001137, 1.562606840307984468 ) ) ;
#5131=CARTESIAN_POINT ( 'NONE',  ( -21.61293655684001536, -39.20140427513058512, 1.382017864820032971 ) ) ;
#5134=CARTESIAN_POINT ( 'NONE',  ( -23.28248557872775137, -37.50000000000000711, 6.717514421272141156 ) ) ;
#5141=CARTESIAN_POINT ( 'NONE',  ( -23.71967171589458445, -49.74859572486944614, -6.359104887540838469 ) ) ;
#5142=CARTESIAN_POINT ( 'NONE',  ( -38.87487832006816291, -31.85140427513056594, -4.584493831696867971 ) ) ;
#5144=CARTESIAN_POINT ( 'NONE',  ( -25.63988726744978663, -32.60140427513057659, -8.440510857627391061 ) ) ;
#5154=CARTESIAN_POINT ( 'NONE',  ( -33.85891924778610473, -47.10000000000000142, 7.573555455601171715 ) ) ;
#5168=CARTESIAN_POINT ( 'NONE',  ( -21.18131961722757595, -47.04859572486944330, -1.453139578080854699 ) ) ;
#5170=CARTESIAN_POINT ( 'NONE',  ( -34.31290974752564438, -32.10000000000000142, 8.464561979789547053 ) ) ;
#5171=CARTESIAN_POINT ( 'NONE',  ( -23.64089511245930098, -38.75140427513058228, -6.280328284105564762 ) ) ;
#5174=CARTESIAN_POINT ( 'NONE',  ( -36.75497492228666374, -39.99859572486943904, -6.680053920257780220 ) ) ;
#5175=CARTESIAN_POINT ( 'NONE',  ( -28.51387258211773812, -34.80000000000000426, 9.383039235653802379 ) ) ;
#5176=CARTESIAN_POINT ( 'NONE',  ( -36.01040764008574513, -30.00000000000000711, -6.010407640085605685 ) ) ;
#5181=CARTESIAN_POINT ( 'NONE',  ( -38.40363834695740053, -48.69859572486944188, -1.277368040863739118 ) ) ;
#5182=CARTESIAN_POINT ( 'NONE',  ( -21.09983283352784156, -49.35000000000000853, 4.534861676072186043 ) ) ;
#5185=CARTESIAN_POINT ( 'NONE',  ( -31.43380250590416125, -35.30140427513057944, -9.391326687552492558 ) ) ;
#5191=CARTESIAN_POINT ( 'NONE',  ( -37.57355545560112375, -38.40000000000000568, 3.858919247786223305 ) ) ;
#5196=CARTESIAN_POINT ( 'NONE',  ( -21.61293655684001536, -36.20140427513057091, 1.382017864820032971 ) ) ;
#5200=CARTESIAN_POINT ( 'NONE',  ( -31.32969295284206979, -36.30000000000000426, -8.395350895058669494 ) ) ;
#5203=CARTESIAN_POINT ( 'NONE',  ( -39.38303923565386100, -47.70000000000000284, -1.486127417882099788 ) ) ;
#5206=CARTESIAN_POINT ( 'NONE',  ( -26.18828373723858149, -49.59859572486944046, -7.597606577763319713 ) ) ;
#5207=CARTESIAN_POINT ( 'NONE',  ( -31.48612741788231517, -36.30000000000000426, -9.383039235653804155 ) ) ;
#5208=CARTESIAN_POINT ( 'NONE',  ( -28.54686042191934092, -35.45140427513057801, -8.818680382772479120 ) ) ;
#5213=CARTESIAN_POINT ( 'NONE',  ( -25.41550616830297571, -41.64859572486943762, 8.874878320068054549 ) ) ;
#5214=CARTESIAN_POINT ( 'NONE',  ( -22.93678734525658314, -39.74999999999999289, -7.063212654743582952 ) ) ;
#5220=CARTESIAN_POINT ( 'NONE',  ( -25.89286002894218086, -50.64859572486944472, 7.938018618334153231 ) ) ;
#5221=CARTESIAN_POINT ( 'NONE',  ( -34.48522952044771017, -35.15140427513058086, -8.925456012876139766 ) ) ;
#5223=CARTESIAN_POINT ( 'NONE',  ( -28.56619749409589204, -33.80140427513056522, 9.391326687552490782 ) ) ;
#5231=CARTESIAN_POINT ( 'NONE',  ( -38.82739432537914581, -38.54999999999999716, 1.398121909749243441 ) ) ;
#5237=CARTESIAN_POINT ( 'NONE',  ( -20.61696076434619584, -43.20000000000000995, 1.486127417882100676 ) ) ;
#5241=CARTESIAN_POINT ( 'NONE',  ( -33.90612223281073057, -34.10140427513057659, 7.549504333439023718 ) ) ;
#5243=CARTESIAN_POINT ( 'NONE',  ( -31.39812190974910422, -31.95000000000000639, 8.827394325379140483 ) ) ;
#5248=CARTESIAN_POINT ( 'NONE',  ( -28.61798213517984024, -50.79859572486945041, 8.387063443159973986 ) ) ;
#5249=CARTESIAN_POINT ( 'NONE',  ( -37.06321265474346660, -38.25000000000001421, 7.063212654743582952 ) ) ;
#5250=CARTESIAN_POINT ( 'NONE',  ( -21.16389173201424612, -42.05140427513057944, -1.343104241417630185 ) ) ;
#5253=CARTESIAN_POINT ( 'NONE',  ( -20.60867331244750034, -38.19859572486942767, 1.433802505903951419 ) ) ;
#5254=CARTESIAN_POINT ( 'NONE',  ( -31.48612741788231517, -42.30000000000000426, -9.383039235653804155 ) ) ;
#5260=CARTESIAN_POINT ( 'NONE',  ( -28.65689575858256077, -49.44859572486943478, -8.836108267985801845 ) ) ;
#5261=CARTESIAN_POINT ( 'NONE',  ( -21.51138689804841420, -35.90140427513058086, -4.265706762501151772 ) ) ;
#5264=CARTESIAN_POINT ( 'NONE',  ( -38.48861310195163554, -46.40140427513058086, 4.265706762501153548 ) ) ;
#5271=CARTESIAN_POINT ( 'NONE',  ( -34.05750781543318340, -42.15000000000001279, -7.963307464738195840 ) ) ;
#5275=CARTESIAN_POINT ( 'NONE',  ( -25.46513832392765408, -43.64999999999999147, 8.900167166472096270 ) ) ;
#5278=CARTESIAN_POINT ( 'NONE',  ( -31.45313957808072303, -30.95140427513058157, 8.818680382772479120 ) ) ;
#5280=CARTESIAN_POINT ( 'NONE',  ( -38.82739432537914581, -32.55000000000000426, 1.398121909749243663 ) ) ;
#5283=CARTESIAN_POINT ( 'NONE',  ( -28.51387258211773812, -46.80000000000001137, 9.383039235653802379 ) ) ;
#5288=CARTESIAN_POINT ( 'NONE',  ( -31.48612741788231517, -48.30000000000001137, -9.383039235653804155 ) ) ;
#5289=CARTESIAN_POINT ( 'NONE',  ( -31.32969295284206979, -30.30000000000000782, -8.395350895058669494 ) ) ;
#5293=CARTESIAN_POINT ( 'NONE',  ( -28.49241082802385350, -40.44859572486944188, -9.874625247442173404 ) ) ;
#5302=CARTESIAN_POINT ( 'NONE',  ( -37.54950433343896776, -33.39859572486943762, 3.906122232810848249 ) ) ;
#5303=CARTESIAN_POINT ( 'NONE',  ( -23.71967171589458445, -46.74859572486943904, -6.359104887540838469 ) ) ;
#5304=CARTESIAN_POINT ( 'NONE',  ( -38.46456197978948666, -50.40000000000000568, 4.312909747525784709 ) ) ;
#5309=CARTESIAN_POINT ( 'NONE',  ( -22.89739904353894318, -47.75140427513058938, -7.023824353025938549 ) ) ;
#5316=CARTESIAN_POINT ( 'NONE',  ( -22.42644454439892598, -39.90000000000000568, -3.858919247786222861 ) ) ;
#5322=CARTESIAN_POINT ( 'NONE',  ( -31.56260684030781505, -43.95000000000000284, 9.865911304835510265 ) ) ;
#5326=CARTESIAN_POINT ( 'NONE',  ( -21.16389173201424612, -33.05140427513057233, -1.343104241417630185 ) ) ;
#5328=CARTESIAN_POINT ( 'NONE',  ( -31.39812190974910422, -37.94999999999999574, 8.827394325379140483 ) ) ;
#5330=CARTESIAN_POINT ( 'NONE',  ( -31.48612741788231517, -48.30000000000001137, -9.383039235653804155 ) ) ;
#5333=CARTESIAN_POINT ( 'NONE',  ( -22.93678734525658314, -45.74999999999999289, -7.063212654743582952 ) ) ;
#5334=CARTESIAN_POINT ( 'NONE',  ( -22.42644454439892598, -30.90000000000000924, -3.858919247786222861 ) ) ;
#5337=CARTESIAN_POINT ( 'NONE',  ( -31.53845232986046554, -40.29859572486944330, -9.374751783755117529 ) ) ;
#5344=CARTESIAN_POINT ( 'NONE',  ( -38.40363834695740053, -33.69859572486942767, -1.277368040863739118 ) ) ;
#5345=CARTESIAN_POINT ( 'NONE',  ( -28.46154767013959486, -41.79859572486943620, 9.374751783755112200 ) ) ;
#5346=CARTESIAN_POINT ( 'NONE',  ( -20.12537475255788522, -39.05140427513057944, -1.507589171976365439 ) ) ;
#5350=CARTESIAN_POINT ( 'NONE',  ( -39.87462524744216807, -49.55140427513056522, 1.507589171976367215 ) ) ;
#5358=CARTESIAN_POINT ( 'NONE',  ( -36.01040764008574513, -48.00000000000000711, -6.010407640085605685 ) ) ;
#5359=CARTESIAN_POINT ( 'NONE',  ( -20.13408869516453947, -37.05000000000001137, -1.562606840307983136 ) ) ;
#5364=CARTESIAN_POINT ( 'NONE',  ( -21.09983283352784156, -40.35000000000000142, 4.534861676072186043 ) ) ;
#5367=CARTESIAN_POINT ( 'NONE',  ( -35.97294713907137975, -35.00140427513057517, -6.047868141099968398 ) ) ;
#5370=CARTESIAN_POINT ( 'NONE',  ( -38.39535089505872634, -38.70000000000000284, -1.329692952841885267 ) ) ;
#5376=CARTESIAN_POINT ( 'NONE',  ( -38.90016716647221529, -47.85000000000000853, -4.534861676072185155 ) ) ;
#5377=CARTESIAN_POINT ( 'NONE',  ( -22.06198138166579170, -45.35140427513057659, 4.107139971057695682 ) ) ;
#5381=CARTESIAN_POINT ( 'NONE',  ( -28.49241082802385350, -46.44859572486943478, -9.874625247442173404 ) ) ;
#5388=CARTESIAN_POINT ( 'NONE',  ( -38.39535089505872634, -47.70000000000000284, -1.329692952841885267 ) ) ;
#5389=CARTESIAN_POINT ( 'NONE',  ( -38.92545601287626056, -42.84859572486944046, -4.485229520447501450 ) ) ;
#5390=CARTESIAN_POINT ( 'NONE',  ( -25.63988726744978663, -41.60140427513058370, -8.440510857627391061 ) ) ;
#5394=CARTESIAN_POINT ( 'NONE',  ( -34.48522952044771017, -41.15140427513058086, -8.925456012876139766 ) ) ;
#5401=CARTESIAN_POINT ( 'NONE',  ( -23.71967171589458445, -31.74859572486943193, -6.359104887540838469 ) ) ;
#5402=CARTESIAN_POINT ( 'NONE',  ( -38.90016716647221529, -32.85000000000000853, -4.534861676072185155 ) ) ;
#5408=CARTESIAN_POINT ( 'NONE',  ( -28.51387258211773812, -40.80000000000000426, 9.383039235653802379 ) ) ;
#5411=CARTESIAN_POINT ( 'NONE',  ( -23.64089511245930098, -47.75140427513058938, -6.280328284105564762 ) ) ;
#5415=CARTESIAN_POINT ( 'NONE',  ( -22.42644454439892598, -48.90000000000000568, -3.858919247786222861 ) ) ;
#5421=CARTESIAN_POINT ( 'NONE',  ( -28.43739315969223824, -45.45000000000000995, -9.865911304835512041 ) ) ;
#5422=CARTESIAN_POINT ( 'NONE',  ( -35.97294713907137975, -50.00140427513058938, -6.047868141099968398 ) ) ;
#5426=AXIS2_PLACEMENT_3D ( 'NONE', #5656, #1649, #2897 ) ;
#5428=CARTESIAN_POINT ( 'NONE',  ( -39.85719736222883824, -45.54859572486944330, 1.617624508639602388 ) ) ;
#5433=CARTESIAN_POINT ( 'NONE',  ( -28.65689575858256077, -31.44859572486944188, -8.836108267985801845 ) ) ;
#5434=CARTESIAN_POINT ( 'NONE',  ( -38.44051085762733777, -36.39859572486944472, 4.360112732550414982 ) ) ;
#5435=CARTESIAN_POINT ( 'NONE',  ( -21.12512167993187973, -39.35140427513057659, 4.584493831696868860 ) ) ;
#5438=CARTESIAN_POINT ( 'NONE',  ( -21.51138689804841420, -44.90140427513058086, -4.265706762501151772 ) ) ;
#5445=CARTESIAN_POINT ( 'NONE',  ( -38.39535089505872634, -47.70000000000000284, -1.329692952841885267 ) ) ;
#5446=CARTESIAN_POINT ( 'NONE',  ( -36.71751442127229836, -39.00000000000000711, -6.717514421272142044 ) ) ;
#5456=CARTESIAN_POINT ( 'NONE',  ( -37.59760657776328685, -40.40140427513058086, 3.811716262761598362 ) ) ;
#5459=UNCERTAINTY_MEASURE_WITH_UNIT (LENGTH_MEASURE( 1.000000000000000082E-05 ), #974, 'distance_accuracy_value', 'NONE');
#5460=CARTESIAN_POINT ( 'NONE',  ( -36.31971658582311591, -41.25000000000000711, 6.319716585823200283 ) ) ;
#5465=CARTESIAN_POINT ( 'NONE',  ( -20.61696076434619584, -49.20000000000000995, 1.486127417882100676 ) ) ;
#5466=CARTESIAN_POINT ( 'NONE',  ( -21.61293655684001536, -45.20140427513059223, 1.382017864820032971 ) ) ;
#5470=CARTESIAN_POINT ( 'NONE',  ( -31.53845232986046554, -46.29859572486944330, -9.374751783755117529 ) ) ;
#5472=CARTESIAN_POINT ( 'NONE',  ( -28.51387258211773812, -34.80000000000000426, 9.383039235653802379 ) ) ;
#5476=CARTESIAN_POINT ( 'NONE',  ( -23.95213185889994989, -32.49859572486943904, 5.972947139071243861 ) ) ;
#5479=CARTESIAN_POINT ( 'NONE',  ( -23.24502507771338600, -41.49859572486943904, 6.680053920257780220 ) ) ;
#5480=CARTESIAN_POINT ( 'NONE',  ( -21.12512167993187973, -42.35140427513057659, 4.584493831696868860 ) ) ;
#5492=CARTESIAN_POINT ( 'NONE',  ( -23.68028341417693738, -48.75000000000001421, -6.319716585823198507 ) ) ;
#5493=CARTESIAN_POINT ( 'NONE',  ( -34.53486167607238144, -33.15000000000001279, -8.900167166472096270 ) ) ;
#5495=CARTESIAN_POINT ( 'NONE',  ( -34.53486167607238144, -45.14999999999999858, -8.900167166472096270 ) ) ;
#5500=CARTESIAN_POINT ( 'NONE',  ( -39.38303923565386100, -50.70000000000000995, -1.486127417882099788 ) ) ;
#5503=CARTESIAN_POINT ( 'NONE',  ( -31.27736804086391942, -47.30140427513057944, -8.403638346957361449 ) ) ;
#5507=CARTESIAN_POINT ( 'NONE',  ( -28.67030704715798350, -43.80000000000000426, 8.395350895058669494 ) ) ;
#5514=CARTESIAN_POINT ( 'NONE',  ( -23.68028341417693738, -36.75000000000000711, -6.319716585823198507 ) ) ;
#5515=( BOUNDED_CURVE ( )  B_SPLINE_CURVE ( 2, ( #977, #3673, #8438, #5079, #3022, #5695, #7063, #3321, #6697, #7274, #2523, #7188, #4678, #5243, #2570, #1147, #7940, #5280, #3974, #3842, #4019, #5994, #7987, #1904, #3229, #4590, #4545, #7231, #8686, #1863, #1234, #5912, #7320, #1990, #6524, #1191, #2659, #2701, #3364, #1946, #7365, #8602, #5200, #3275, #6566, #473, #4631, #3931, #8560, #3886, #1273, #7896, #6607, #5328, #8076, #609, #6653, #519, #5370, #8030, #1319, #562, #3188, #5868, #657, #6038, #1144, #8647, #5954, #4501, #2613, #2173, #4107, #4903, #7408, #5460, #2834, #4861, #4812, #6741, #5553, #8168, #1366, #2131, #2083, #43, #4724, #2220, #2793, #91, #4065, #7496, #5507, #1498, #702, #1543, #8217, #7453, #2925, #1458, #4152, #4768, #1410, #6218, #8124, #6830, #748, #7537, #8259, #3407, #6785, #3540, #223, #882, #4193, #7582, #795, #3497, #6176, #6875, #5599, #837, #134, #6086, #3454, #182, #5415, #2880, #4238, #2036, #6918, #3583, #6130, #2747, #6265, #8431, #3710, #1102, #4989, #3915, #266 ),
 .UNSPECIFIED., .F., .T. ) 
 B_SPLINE_CURVE_WITH_KNOTS ( ( 3, 2, 2, 2, 2, 2, 2, 2, 2, 2, 2, 2, 2, 2, 2, 2, 2, 2, 2, 2, 2, 2, 2, 2, 2, 2, 2, 2, 2, 2, 2, 2, 2, 2, 2, 2, 2, 2, 2, 2, 2, 2, 2, 2, 2, 2, 2, 2, 2, 2, 2, 2, 2, 2, 2, 2, 2, 2, 2, 2, 2, 2, 2, 2, 2, 2, 2, 2, 2, 2, 3 ),
 ( 0.000000000000000000, 0.01428571428571428527, 0.02857142857142857054, 0.04285714285714285754, 0.05714285714285714107, 0.07142857142857142461, 0.08571428571428571508, 0.1000000000000000056, 0.1142857142857142821, 0.1285714285714285587, 0.1428571428571428492, 0.1571428571428571397, 0.1714285714285714302, 0.1857142857142857206, 0.2000000000000000111, 0.2142857142857142738, 0.2285714285714285643, 0.2428571428571428548, 0.2571428571428571175, 0.2714285714285714080, 0.2857142857142856984, 0.2999999999999999889, 0.3142857142857142794, 0.3285714285714285698, 0.3428571428571428603, 0.3571428571428571508, 0.3714285714285714413, 0.3857142857142857317, 0.4000000000000000222, 0.4142857142857143127, 0.4285714285714285476, 0.4428571428571428381, 0.4571428571428571286, 0.4714285714285714191, 0.4857142857142857095, 0.5000000000000000000, 0.5142857142857142350, 0.5285714285714285809, 0.5428571428571428159, 0.5571428571428571619, 0.5714285714285713969, 0.5857142857142857428, 0.5999999999999999778, 0.6142857142857143238, 0.6285714285714285587, 0.6428571428571429047, 0.6571428571428571397, 0.6714285714285713746, 0.6857142857142857206, 0.6999999999999999556, 0.7142857142857143016, 0.7285714285714285365, 0.7428571428571428825, 0.7571428571428571175, 0.7714285714285714635, 0.7857142857142856984, 0.8000000000000000444, 0.8142857142857142794, 0.8285714285714286254, 0.8428571428571428603, 0.8571428571428570953, 0.8714285714285714413, 0.8857142857142856762, 0.9000000000000000222, 0.9142857142857142572, 0.9285714285714286031, 0.9428571428571428381, 0.9571428571428571841, 0.9714285714285714191, 0.9857142857142857650, 1.000000000000000000 ),
 .UNSPECIFIED. ) 
 CURVE ( )  GEOMETRIC_REPRESENTATION_ITEM ( )  RATIONAL_B_SPLINE_CURVE ( ( 1.000000000000000000, 0.9510565162951535312, 1.000000000000000000, 0.9510565162951535312, 1.000000000000000000, 0.9510565162951535312, 1.000000000000000000, 0.9510565162951535312, 1.000000000000000000, 0.9510565162951535312, 1.000000000000000000, 0.9510565162951535312, 1.000000000000000000, 0.9510565162951535312, 1.000000000000000000, 0.9510565162951535312, 1.000000000000000000, 0.9510565162951535312, 1.000000000000000000, 0.9510565162951535312, 1.000000000000000000, 0.9510565162951535312, 1.000000000000000000, 0.9510565162951535312, 1.000000000000000000, 0.9510565162951535312, 1.000000000000000000, 0.9510565162951535312, 1.000000000000000000, 0.9510565162951535312, 1.000000000000000000, 0.9510565162951535312, 1.000000000000000000, 0.9510565162951535312, 1.000000000000000000, 0.9510565162951535312, 1.000000000000000000, 0.9510565162951535312, 1.000000000000000000, 0.9510565162951535312, 1.000000000000000000, 0.9510565162951535312, 1.000000000000000000, 0.9510565162951535312, 1.000000000000000000, 0.9510565162951535312, 1.000000000000000000, 0.9510565162951535312, 1.000000000000000000, 0.9510565162951535312, 1.000000000000000000, 0.9510565162951535312, 1.000000000000000000, 0.9510565162951535312, 1.000000000000000000, 0.9510565162951535312, 1.000000000000000000, 0.9510565162951535312, 1.000000000000000000, 0.9510565162951535312, 1.000000000000000000, 0.9510565162951535312, 1.000000000000000000, 0.9510565162951535312, 1.000000000000000000, 0.9510565162951535312, 1.000000000000000000, 0.9510565162951535312, 1.000000000000000000, 0.9510565162951535312, 1.000000000000000000, 0.9510565162951535312, 1.000000000000000000, 0.9510565162951535312, 1.000000000000000000, 0.9510565162951535312, 1.000000000000000000, 0.9510565162951535312, 1.000000000000000000, 0.9510565162951535312, 1.000000000000000000, 0.9510565162951535312, 1.000000000000000000, 0.9510565162951535312, 1.000000000000000000, 0.9510565162951535312, 1.000000000000000000, 0.9510565162951535312, 1.000000000000000000, 0.9510565162951535312, 1.000000000000000000, 0.9510565162951535312, 1.000000000000000000, 0.9510565162951535312, 1.000000000000000000, 0.9510565162951535312, 1.000000000000000000, 0.9510565162951535312, 1.000000000000000000, 0.9510565162951535312, 1.000000000000000000, 0.9510565162951535312, 1.000000000000000000, 0.9510565162951535312, 1.000000000000000000, 0.9510565162951535312, 1.000000000000000000, 0.9510565162951535312, 1.000000000000000000, 0.9510565162951535312, 1.000000000000000000, 0.9510565162951535312, 1.000000000000000000, 0.9510565162951535312, 1.000000000000000000, 0.9510565162951535312, 1.000000000000000000, 0.9510565162951535312, 1.000000000000000000, 0.9510565162951535312, 1.000000000000000000, 0.9510565162951535312, 1.000000000000000000, 0.9510565162951535312, 1.000000000000000000, 0.9510565162951535312, 1.000000000000000000, 0.9510565162951535312, 1.000000000000000000, 0.9510565162951535312, 1.000000000000000000, 0.9510565162951535312, 1.000000000000000000, 0.9510565162951535312, 1.000000000000000000, 0.9510565162951535312, 1.000000000000000000, 0.9510565162951535312, 1.000000000000000000, 0.9510565162951535312, 1.000000000000000000 ) ) 
 REPRESENTATION_ITEM ( '' )  );
#5519=CARTESIAN_POINT ( 'NONE',  ( -21.07454398712378918, -50.34859572486944046, 4.485229520447505003 ) ) ;
#5527=CARTESIAN_POINT ( 'NONE',  ( -38.40363834695740053, -39.69859572486944188, -1.277368040863739118 ) ) ;
#5528=CARTESIAN_POINT ( 'NONE',  ( -38.92545601287626056, -36.84859572486944046, -4.485229520447501450 ) ) ;
#5529=CARTESIAN_POINT ( 'NONE',  ( -34.36011273255026310, -43.10140427513058370, 8.440510857627391061 ) ) ;
#5539=CARTESIAN_POINT ( 'NONE',  ( -38.40363834695740053, -36.69859572486944188, -1.277368040863739118 ) ) ;
#5540=CARTESIAN_POINT ( 'NONE',  ( -37.06321265474346660, -32.25000000000000711, 7.063212654743582952 ) ) ;
#5542=CARTESIAN_POINT ( 'NONE',  ( -21.53543802021056663, -48.90000000000000568, -4.312909747525783821 ) ) ;
#5549=CARTESIAN_POINT ( 'NONE',  ( -33.90612223281073057, -40.10140427513057659, 7.549504333439023718 ) ) ;
#5551=UNCERTAINTY_MEASURE_WITH_UNIT (LENGTH_MEASURE( 1.000000000000000082E-05 ), #7150, 'distance_accuracy_value', 'NONE');
#5553=CARTESIAN_POINT ( 'NONE',  ( -36.01040764008574513, -42.00000000000000711, -6.010407640085605685 ) ) ;
#5557=CARTESIAN_POINT ( 'NONE',  ( -31.32969295284206979, -42.30000000000000426, -8.395350895058669494 ) ) ;
#5560=CARTESIAN_POINT ( 'NONE',  ( -37.02382435302582309, -45.24859572486943904, 7.102600956461226467 ) ) ;
#5566=CARTESIAN_POINT ( 'NONE',  ( -23.71967171589458445, -43.74859572486943904, -6.359104887540838469 ) ) ;
#5567=CARTESIAN_POINT ( 'NONE',  ( -21.55948914237271907, -46.89859572486944472, -4.360112732550413206 ) ) ;
#5568=CARTESIAN_POINT ( 'NONE',  ( -22.40239342223677355, -29.90140427513058796, -3.811716262761597473 ) ) ;
#5569=( BOUNDED_SURFACE ( )  B_SPLINE_SURFACE ( 3, 2, ( 
 ( #168, #4140, #6905, #6204, #6819, #1485, #3526, #6166, #2732, #2690, #2024, #122, #2070, #4890, #2866, #5540, #8158, #73, #8246, #5402, #6862, #5493, #7441, #8203, #4052, #1399, #781, #3353, #2821, #6073, #691, #2205, #3484, #2161, #4847, #7567, #7526, #4180, #1352, #6029, #1528, #4095, #6732, #826, #4222, #2117, #7768, #5359, #8061, #4714, #31, #7397, #2781, #6771, #3397, #8111, #4756, #736, #3441, #6118, #5446, #4800, #7482, #1446, #3568, #6290, #2997, #2249, #7657, #6331, #2292, #7611, #8376, #2954, #209, #7037, #295, #4928, #914, #3695, #4267, #5672, #8418, #4442, #5717, #336, #6950, #1760, #997, #6375, #6253, #252, #1045, #8289, #1573, #5582, #3609, #5628, #8328, #1665, #2336, #8458, #375, #5017, #2912, #7706, #1711, #5760, #4974, #6993, #1619, #957, #4310, #3653, #4357, #3042, #867, #2382, #4398, #5057, #7747, #7087, #3737, #6418, #3083, #7791, #2421, #5101, #1922, #5182, #5804, #412, #8578, #7250, #1964, #1842, #5304, #1086, #1799, #1212, #5893 ),
 ( #6585, #4481, #8007, #4568, #3907, #3783, #3820, #7295, #8498, #7834, #3124, #7167, #6500, #2460, #7919, #6543, #5974, #6626, #3866, #5142, #2544, #7960, #3300, #3170, #4523, #6460, #7209, #1127, #1170, #453, #5846, #7125, #494, #4610, #1883, #3208, #8537, #540, #3251, #7876, #2504, #5221, #5931, #1252, #8624, #2592, #5261, #3950, #584, #8666, #2633, #4039, #3995, #3339, #7470, #3383, #6193, #1475, #7514, #721, #1386, #6850, #6719, #8189, #6808, #19, #769, #5346, #2720, #5435, #4652, #1431, #7386, #2011, #4169, #2105, #3472, #4127, #815, #6153, #111, #2677, #7339, #4835, #5390, #8049, #2809, #4787, #3429, #5480, #1295, #3516, #8145, #1340, #5529, #4082, #8099, #2149, #156, #2853, #4701, #8233, #6675, #678, #631, #6017, #8705, #6059, #2057, #6758, #4743, #7429, #6103, #63, #2767, #7598, #8363, #7025, #4345, #7075, #239, #1607, #7555, #4918, #986, #3684, #5703, #6322, #1562, #6239, #1518, #3600, #6364, #6280, #6893, #4297, #3726, #4211, #3072, #6408, #2942 ),
 ( #2901, #856, #5617, #945, #285, #8318, #5568, #8275, #5749, #3555, #6981, #1698, #3641, #2986, #1034, #2281, #326, #199, #5661, #7736, #2192, #2326, #5004, #7692, #1653, #363, #3032, #8406, #4962, #902, #7644, #2239, #4256, #2370, #6939, #5046, #4388, #4878, #6573, #1241, #526, #6489, #4431, #5208, #3110, #401, #7196, #7863, #1156, #8567, #3284, #3159, #6615, #2409, #5790, #2531, #3850, #2450, #8523, #5919, #7822, #570, #8447, #5088, #6449, #5171, #8485, #1075, #5131, #7778, #5878, #3237, #4598, #6532, #480, #5834, #440, #3937, #3195, #2580, #1748, #2489, #7904, #1871, #1828, #7113, #8609, #5250, #4554, #3768, #7947, #7282, #1787, #4469, #7154, #7238, #1115, #3807, #4509, #1198, #3894, #1910, #665, #6661, #617, #804, #7326, #8085, #5466, #5377, #4071, #4819, #6704, #1419, #4638, #2043, #2797, #5961, #4731, #7416, #2755, #1374, #7502, #7460, #710, #3371, #4687, #6045, #6002, #8693, #4114, #3328, #6747, #3982, #2666, #6793, #1463, #757, #4027, #1953, #5422 ),
 ( #3415, #8037, #5289, #6093, #2708, #1281, #5334, #51, #2620, #7, #3460, #1997, #6836, #8655, #7995, #7372, #8132, #1326, #2092, #4775, #6138, #98, #8175, #2138, #4158, #2269, #887, #4242, #7725, #4285, #6352, #142, #6924, #6967, #3628, #6268, #8223, #7012, #314, #934, #7059, #3018, #2356, #5035, #2841, #5514, #270, #3504, #185, #6309, #8348, #5648, #8393, #1547, #2929, #2180, #6224, #2314, #4992, #975, #7629, #2888, #7542, #4867, #4905, #7675, #7587, #1505, #5603, #1684, #4200, #4374, #6182, #3588, #6880, #843, #5693, #1640, #2972, #4333, #3670, #1592, #5557, #3544, #8263, #227, #2225, #8306, #4948, #5738, #4419, #1020, #3713, #6396, #8435, #352, #3060, #2398, #5075, #7765, #1733, #5971, #2009, #8097, #4741, #4036, #1292, #3993, #4167, #1962, #2718, #109, #17, #7427, #8187, #1338, #4785, #8005, #5388, #6151, #582, #2055, #1384, #6101, #4080, #2147, #2102, #6756, #6717, #8047, #675, #628, #3337, #7468, #6673, #719, #7337, #6015, #1429, #4833, #4125 ),
 ( #3427, #61, #2765, #5433, #3298, #3381, #7512, #8664, #8703, #6057, #5476, #2631, #7384, #6806, #2675, #1473, #5302, #4650, #5344, #8143, #4699, #767, #3470, #2807, #4295, #1651, #3030, #2279, #5615, #4254, #7596, #2368, #7642, #984, #3514, #1559, #1605, #6978, #900, #2851, #4343, #3681, #943, #1696, #6361, #5701, #8404, #6191, #153, #3639, #6848, #3553, #6320, #2984, #283, #5044, #4916, #6277, #5527, #854, #5658, #2899, #6937, #8231, #3598, #2190, #237, #6890, #4876, #813, #2940, #7023, #8361, #8316, #7553, #2324, #5002, #4959, #7734, #1516, #6237, #324, #7689, #4209, #197, #5566, #8273, #2236, #7194, #3765, #3724, #3070, #1153, #3108, #5917, #1196, #7236, #437, #1113, #6571, #6447, #7902, #6530, #8482, #478, #5086, #2448, #5168, #4386, #3848, #7111, #1746, #3892, #1826, #3193, #5876, #524, #8565, #2529, #2407, #7072, #4552, #5129, #7775, #5206, #4507, #3157, #1868, #1032, #3235, #7861, #1073, #5248, #3805, #7820, #8607, #2577, #7945, #4429, #6406, #361 ),
 ( #1785, #5747, #8445, #399, #5788, #5832, #6487, #8521, #4467, #7152, #2487, #573, #1956, #574, #2001, #6618, #1285, #5965, #7158, #3289, #8658, #1831, #8040, #4602, #7285, #3811, #3856, #7330, #5837, #7867, #3163, #4513, #6535, #8527, #7951, #6576, #6007, #6665, #3898, #444, #2583, #7999, #3330, #1161, #6493, #1244, #4642, #8696, #5253, #5923, #4559, #7908, #2669, #1914, #3985, #2493, #1874, #3941, #2624, #1203, #5174, #621, #5337, #5293, #1118, #7200, #484, #3200, #5883, #8570, #2534, #5213, #7242, #530, #3241, #8614, #847, #2758, #4118, #1329, #7422, #3508, #6185, #8227, #103, #1377, #11, #4031, #6096, #6840, #55, #669, #6799, #6228, #6709, #5560, #190, #5428, #7378, #2891, #1510, #146, #5470, #5381, #3374, #8137, #3463, #2800, #2096, #8090, #2047, #8267, #6049, #760, #4203, #6144, #8179, #3547, #4778, #2844, #2711, #2142, #6884, #4692, #4824, #7505, #1467, #4160, #4735, #5519, #807, #7464, #3420, #1423, #4074, #6751, #2183, #713, #4871, #7546, #8309 ),
 ( #7729, #5606, #2933, #978, #1644, #3674, #2360, #5907, #3592, #5038, #4909, #892, #4996, #7107, #7590, #274, #8439, #1597, #3225, #2230, #1552, #230, #7680, #2272, #6271, #4246, #2317, #4953, #7633, #6928, #4336, #5742, #3023, #7015, #4288, #8398, #1689, #2976, #513, #6972, #937, #2403, #5652, #3631, #6313, #5696, #357, #5080, #4379, #8353, #6355, #318, #7064, #1025, #3881, #7770, #1739, #3718, #6401, #4423, #3065, #1068, #6560, #3967, #2030, #555, #6644, #649, #8595, #5364, #2607, #5947, #5408, #6033, #4718, #8067, #2075, #7402, #2696, #6600, #2560, #36, #601, #3267, #1357, #4951, #7358, #4057, #5237, #8117, #3358, #5275, #742, #5322, #3315, #695, #6736, #3401, #8641, #6078, #2739, #7979, #4762, #7446, #1404, #7932, #1941, #1983, #1228, #5989, #8022, #1267, #4626, #1312, #7310, #8680, #4012, #6777, #4100, #3447, #1899, #4583, #7267, #3925, #2653, #4670, #6691, #788, #7001, #3576, #6260, #2786, #2827, #6297, #4806, #6824, #2123, #3490, #5500, #7488, #6912 ) ),
 .UNSPECIFIED., .T., .F., .T. ) 
 B_SPLINE_SURFACE_WITH_KNOTS ( ( 4, 3, 4 ),
 ( 3, 2, 2, 2, 2, 2, 2, 2, 2, 2, 2, 2, 2, 2, 2, 2, 2, 2, 2, 2, 2, 2, 2, 2, 2, 2, 2, 2, 2, 2, 2, 2, 2, 2, 2, 2, 2, 2, 2, 2, 2, 2, 2, 2, 2, 2, 2, 2, 2, 2, 2, 2, 2, 2, 2, 2, 2, 2, 2, 2, 2, 2, 2, 2, 2, 2, 2, 2, 2, 2, 3 ),
 ( 0.000000000000000000, 0.5000000000000000000, 1.000000000000000000 ),
 ( 0.000000000000000000, 0.01428571428571428527, 0.02857142857142857054, 0.04285714285714285754, 0.05714285714285714107, 0.07142857142857142461, 0.08571428571428571508, 0.1000000000000000056, 0.1142857142857142821, 0.1285714285714285587, 0.1428571428571428492, 0.1571428571428571397, 0.1714285714285714302, 0.1857142857142857206, 0.2000000000000000111, 0.2142857142857142738, 0.2285714285714285643, 0.2428571428571428548, 0.2571428571428571175, 0.2714285714285714080, 0.2857142857142856984, 0.2999999999999999889, 0.3142857142857142794, 0.3285714285714285698, 0.3428571428571428603, 0.3571428571428571508, 0.3714285714285714413, 0.3857142857142857317, 0.4000000000000000222, 0.4142857142857143127, 0.4285714285714285476, 0.4428571428571428381, 0.4571428571428571286, 0.4714285714285714191, 0.4857142857142857095, 0.5000000000000000000, 0.5142857142857142350, 0.5285714285714285809, 0.5428571428571428159, 0.5571428571428571619, 0.5714285714285713969, 0.5857142857142857428, 0.5999999999999999778, 0.6142857142857143238, 0.6285714285714285587, 0.6428571428571429047, 0.6571428571428571397, 0.6714285714285713746, 0.6857142857142857206, 0.6999999999999999556, 0.7142857142857143016, 0.7285714285714285365, 0.7428571428571428825, 0.7571428571428571175, 0.7714285714285714635, 0.7857142857142856984, 0.8000000000000000444, 0.8142857142857142794, 0.8285714285714286254, 0.8428571428571428603, 0.8571428571428570953, 0.8714285714285714413, 0.8857142857142856762, 0.9000000000000000222, 0.9142857142857142572, 0.9285714285714286031, 0.9428571428571428381, 0.9571428571428571841, 0.9714285714285714191, 0.9857142857142857650, 1.000000000000000000 ),
 .UNSPECIFIED. ) 
 GEOMETRIC_REPRESENTATION_ITEM ( )  RATIONAL_B_SPLINE_SURFACE ( (
 ( 1.000000000000000000, 0.9510565162951535312, 1.000000000000000000, 0.9510565162951535312, 1.000000000000000000, 0.9510565162951535312, 1.000000000000000000, 0.9510565162951535312, 1.000000000000000000, 0.9510565162951535312, 1.000000000000000000, 0.9510565162951535312, 1.000000000000000000, 0.9510565162951535312, 1.000000000000000000, 0.9510565162951535312, 1.000000000000000000, 0.9510565162951535312, 1.000000000000000000, 0.9510565162951535312, 1.000000000000000000, 0.9510565162951535312, 1.000000000000000000, 0.9510565162951535312, 1.000000000000000000, 0.9510565162951535312, 1.000000000000000000, 0.9510565162951535312, 1.000000000000000000, 0.9510565162951535312, 1.000000000000000000, 0.9510565162951535312, 1.000000000000000000, 0.9510565162951535312, 1.000000000000000000, 0.9510565162951535312, 1.000000000000000000, 0.9510565162951535312, 1.000000000000000000, 0.9510565162951535312, 1.000000000000000000, 0.9510565162951535312, 1.000000000000000000, 0.9510565162951535312, 1.000000000000000000, 0.9510565162951535312, 1.000000000000000000, 0.9510565162951535312, 1.000000000000000000, 0.9510565162951535312, 1.000000000000000000, 0.9510565162951535312, 1.000000000000000000, 0.9510565162951535312, 1.000000000000000000, 0.9510565162951535312, 1.000000000000000000, 0.9510565162951535312, 1.000000000000000000, 0.9510565162951535312, 1.000000000000000000, 0.9510565162951535312, 1.000000000000000000, 0.9510565162951535312, 1.000000000000000000, 0.9510565162951535312, 1.000000000000000000, 0.9510565162951535312, 1.000000000000000000, 0.9510565162951535312, 1.000000000000000000, 0.9510565162951535312, 1.000000000000000000, 0.9510565162951535312, 1.000000000000000000, 0.9510565162951535312, 1.000000000000000000, 0.9510565162951535312, 1.000000000000000000, 0.9510565162951535312, 1.000000000000000000, 0.9510565162951535312, 1.000000000000000000, 0.9510565162951535312, 1.000000000000000000, 0.9510565162951535312, 1.000000000000000000, 0.9510565162951535312, 1.000000000000000000, 0.9510565162951535312, 1.000000000000000000, 0.9510565162951535312, 1.000000000000000000, 0.9510565162951535312, 1.000000000000000000, 0.9510565162951535312, 1.000000000000000000, 0.9510565162951535312, 1.000000000000000000, 0.9510565162951535312, 1.000000000000000000, 0.9510565162951535312, 1.000000000000000000, 0.9510565162951535312, 1.000000000000000000, 0.9510565162951535312, 1.000000000000000000, 0.9510565162951535312, 1.000000000000000000, 0.9510565162951535312, 1.000000000000000000, 0.9510565162951535312, 1.000000000000000000, 0.9510565162951535312, 1.000000000000000000, 0.9510565162951535312, 1.000000000000000000, 0.9510565162951535312, 1.000000000000000000, 0.9510565162951535312, 1.000000000000000000, 0.9510565162951535312, 1.000000000000000000, 0.9510565162951535312, 1.000000000000000000, 0.9510565162951535312, 1.000000000000000000, 0.9510565162951535312, 1.000000000000000000, 0.9510565162951535312, 1.000000000000000000, 0.9510565162951535312, 1.000000000000000000, 0.9510565162951535312, 1.000000000000000000, 0.9510565162951535312, 1.000000000000000000, 0.9510565162951535312, 1.000000000000000000, 0.9510565162951535312, 1.000000000000000000),
 ( 0.3333333333333333703, 0.3170188387650512141, 0.3333333333333333703, 0.3170188387650512141, 0.3333333333333333703, 0.3170188387650512141, 0.3333333333333333703, 0.3170188387650512141, 0.3333333333333333703, 0.3170188387650512141, 0.3333333333333333703, 0.3170188387650512141, 0.3333333333333333703, 0.3170188387650512141, 0.3333333333333333703, 0.3170188387650512141, 0.3333333333333333703, 0.3170188387650512141, 0.3333333333333333703, 0.3170188387650512141, 0.3333333333333333703, 0.3170188387650512141, 0.3333333333333333703, 0.3170188387650512141, 0.3333333333333333703, 0.3170188387650512141, 0.3333333333333333703, 0.3170188387650512141, 0.3333333333333333703, 0.3170188387650512141, 0.3333333333333333703, 0.3170188387650512141, 0.3333333333333333703, 0.3170188387650512141, 0.3333333333333333703, 0.3170188387650512141, 0.3333333333333333703, 0.3170188387650512141, 0.3333333333333333703, 0.3170188387650512141, 0.3333333333333333703, 0.3170188387650512141, 0.3333333333333333703, 0.3170188387650512141, 0.3333333333333333703, 0.3170188387650512141, 0.3333333333333333703, 0.3170188387650512141, 0.3333333333333333703, 0.3170188387650512141, 0.3333333333333333703, 0.3170188387650512141, 0.3333333333333333703, 0.3170188387650512141, 0.3333333333333333703, 0.3170188387650512141, 0.3333333333333333703, 0.3170188387650512141, 0.3333333333333333703, 0.3170188387650512141, 0.3333333333333333703, 0.3170188387650512141, 0.3333333333333333703, 0.3170188387650512141, 0.3333333333333333703, 0.3170188387650512141, 0.3333333333333333703, 0.3170188387650512141, 0.3333333333333333703, 0.3170188387650512141, 0.3333333333333333703, 0.3170188387650512141, 0.3333333333333333703, 0.3170188387650512141, 0.3333333333333333703, 0.3170188387650512141, 0.3333333333333333703, 0.3170188387650512141, 0.3333333333333333703, 0.3170188387650512141, 0.3333333333333333703, 0.3170188387650512141, 0.3333333333333333703, 0.3170188387650512141, 0.3333333333333333703, 0.3170188387650512141, 0.3333333333333333703, 0.3170188387650512141, 0.3333333333333333703, 0.3170188387650512141, 0.3333333333333333703, 0.3170188387650512141, 0.3333333333333333703, 0.3170188387650512141, 0.3333333333333333703, 0.3170188387650512141, 0.3333333333333333703, 0.3170188387650512141, 0.3333333333333333703, 0.3170188387650512141, 0.3333333333333333703, 0.3170188387650512141, 0.3333333333333333703, 0.3170188387650512141, 0.3333333333333333703, 0.3170188387650512141, 0.3333333333333333703, 0.3170188387650512141, 0.3333333333333333703, 0.3170188387650512141, 0.3333333333333333703, 0.3170188387650512141, 0.3333333333333333703, 0.3170188387650512141, 0.3333333333333333703, 0.3170188387650512141, 0.3333333333333333703, 0.3170188387650512141, 0.3333333333333333703, 0.3170188387650512141, 0.3333333333333333703, 0.3170188387650512141, 0.3333333333333333703, 0.3170188387650512141, 0.3333333333333333703, 0.3170188387650512141, 0.3333333333333333703, 0.3170188387650512141, 0.3333333333333333703, 0.3170188387650512141, 0.3333333333333333703, 0.3170188387650512141, 0.3333333333333333703, 0.3170188387650512141, 0.3333333333333333703, 0.3170188387650512141, 0.3333333333333333703, 0.3170188387650512141, 0.3333333333333333703, 0.3170188387650512141, 0.3333333333333333703),
 ( 0.3333333333333333703, 0.3170188387650512141, 0.3333333333333333703, 0.3170188387650512141, 0.3333333333333333703, 0.3170188387650512141, 0.3333333333333333703, 0.3170188387650512141, 0.3333333333333333703, 0.3170188387650512141, 0.3333333333333333703, 0.3170188387650512141, 0.3333333333333333703, 0.3170188387650512141, 0.3333333333333333703, 0.3170188387650512141, 0.3333333333333333703, 0.3170188387650512141, 0.3333333333333333703, 0.3170188387650512141, 0.3333333333333333703, 0.3170188387650512141, 0.3333333333333333703, 0.3170188387650512141, 0.3333333333333333703, 0.3170188387650512141, 0.3333333333333333703, 0.3170188387650512141, 0.3333333333333333703, 0.3170188387650512141, 0.3333333333333333703, 0.3170188387650512141, 0.3333333333333333703, 0.3170188387650512141, 0.3333333333333333703, 0.3170188387650512141, 0.3333333333333333703, 0.3170188387650512141, 0.3333333333333333703, 0.3170188387650512141, 0.3333333333333333703, 0.3170188387650512141, 0.3333333333333333703, 0.3170188387650512141, 0.3333333333333333703, 0.3170188387650512141, 0.3333333333333333703, 0.3170188387650512141, 0.3333333333333333703, 0.3170188387650512141, 0.3333333333333333703, 0.3170188387650512141, 0.3333333333333333703, 0.3170188387650512141, 0.3333333333333333703, 0.3170188387650512141, 0.3333333333333333703, 0.3170188387650512141, 0.3333333333333333703, 0.3170188387650512141, 0.3333333333333333703, 0.3170188387650512141, 0.3333333333333333703, 0.3170188387650512141, 0.3333333333333333703, 0.3170188387650512141, 0.3333333333333333703, 0.3170188387650512141, 0.3333333333333333703, 0.3170188387650512141, 0.3333333333333333703, 0.3170188387650512141, 0.3333333333333333703, 0.3170188387650512141, 0.3333333333333333703, 0.3170188387650512141, 0.3333333333333333703, 0.3170188387650512141, 0.3333333333333333703, 0.3170188387650512141, 0.3333333333333333703, 0.3170188387650512141, 0.3333333333333333703, 0.3170188387650512141, 0.3333333333333333703, 0.3170188387650512141, 0.3333333333333333703, 0.3170188387650512141, 0.3333333333333333703, 0.3170188387650512141, 0.3333333333333333703, 0.3170188387650512141, 0.3333333333333333703, 0.3170188387650512141, 0.3333333333333333703, 0.3170188387650512141, 0.3333333333333333703, 0.3170188387650512141, 0.3333333333333333703, 0.3170188387650512141, 0.3333333333333333703, 0.3170188387650512141, 0.3333333333333333703, 0.3170188387650512141, 0.3333333333333333703, 0.3170188387650512141, 0.3333333333333333703, 0.3170188387650512141, 0.3333333333333333703, 0.3170188387650512141, 0.3333333333333333703, 0.3170188387650512141, 0.3333333333333333703, 0.3170188387650512141, 0.3333333333333333703, 0.3170188387650512141, 0.3333333333333333703, 0.3170188387650512141, 0.3333333333333333703, 0.3170188387650512141, 0.3333333333333333703, 0.3170188387650512141, 0.3333333333333333703, 0.3170188387650512141, 0.3333333333333333703, 0.3170188387650512141, 0.3333333333333333703, 0.3170188387650512141, 0.3333333333333333703, 0.3170188387650512141, 0.3333333333333333703, 0.3170188387650512141, 0.3333333333333333703, 0.3170188387650512141, 0.3333333333333333703, 0.3170188387650512141, 0.3333333333333333703, 0.3170188387650512141, 0.3333333333333333703, 0.3170188387650512141, 0.3333333333333333703),
 ( 1.000000000000000000, 0.9510565162951535312, 1.000000000000000000, 0.9510565162951535312, 1.000000000000000000, 0.9510565162951535312, 1.000000000000000000, 0.9510565162951535312, 1.000000000000000000, 0.9510565162951535312, 1.000000000000000000, 0.9510565162951535312, 1.000000000000000000, 0.9510565162951535312, 1.000000000000000000, 0.9510565162951535312, 1.000000000000000000, 0.9510565162951535312, 1.000000000000000000, 0.9510565162951535312, 1.000000000000000000, 0.9510565162951535312, 1.000000000000000000, 0.9510565162951535312, 1.000000000000000000, 0.9510565162951535312, 1.000000000000000000, 0.9510565162951535312, 1.000000000000000000, 0.9510565162951535312, 1.000000000000000000, 0.9510565162951535312, 1.000000000000000000, 0.9510565162951535312, 1.000000000000000000, 0.9510565162951535312, 1.000000000000000000, 0.9510565162951535312, 1.000000000000000000, 0.9510565162951535312, 1.000000000000000000, 0.9510565162951535312, 1.000000000000000000, 0.9510565162951535312, 1.000000000000000000, 0.9510565162951535312, 1.000000000000000000, 0.9510565162951535312, 1.000000000000000000, 0.9510565162951535312, 1.000000000000000000, 0.9510565162951535312, 1.000000000000000000, 0.9510565162951535312, 1.000000000000000000, 0.9510565162951535312, 1.000000000000000000, 0.9510565162951535312, 1.000000000000000000, 0.9510565162951535312, 1.000000000000000000, 0.9510565162951535312, 1.000000000000000000, 0.9510565162951535312, 1.000000000000000000, 0.9510565162951535312, 1.000000000000000000, 0.9510565162951535312, 1.000000000000000000, 0.9510565162951535312, 1.000000000000000000, 0.9510565162951535312, 1.000000000000000000, 0.9510565162951535312, 1.000000000000000000, 0.9510565162951535312, 1.000000000000000000, 0.9510565162951535312, 1.000000000000000000, 0.9510565162951535312, 1.000000000000000000, 0.9510565162951535312, 1.000000000000000000, 0.9510565162951535312, 1.000000000000000000, 0.9510565162951535312, 1.000000000000000000, 0.9510565162951535312, 1.000000000000000000, 0.9510565162951535312, 1.000000000000000000, 0.9510565162951535312, 1.000000000000000000, 0.9510565162951535312, 1.000000000000000000, 0.9510565162951535312, 1.000000000000000000, 0.9510565162951535312, 1.000000000000000000, 0.9510565162951535312, 1.000000000000000000, 0.9510565162951535312, 1.000000000000000000, 0.9510565162951535312, 1.000000000000000000, 0.9510565162951535312, 1.000000000000000000, 0.9510565162951535312, 1.000000000000000000, 0.9510565162951535312, 1.000000000000000000, 0.9510565162951535312, 1.000000000000000000, 0.9510565162951535312, 1.000000000000000000, 0.9510565162951535312, 1.000000000000000000, 0.9510565162951535312, 1.000000000000000000, 0.9510565162951535312, 1.000000000000000000, 0.9510565162951535312, 1.000000000000000000, 0.9510565162951535312, 1.000000000000000000, 0.9510565162951535312, 1.000000000000000000, 0.9510565162951535312, 1.000000000000000000, 0.9510565162951535312, 1.000000000000000000, 0.9510565162951535312, 1.000000000000000000, 0.9510565162951535312, 1.000000000000000000, 0.9510565162951535312, 1.000000000000000000, 0.9510565162951535312, 1.000000000000000000, 0.9510565162951535312, 1.000000000000000000),
 ( 0.3333333333333333703, 0.3170188387650512141, 0.3333333333333333703, 0.3170188387650512141, 0.3333333333333333703, 0.3170188387650512141, 0.3333333333333333703, 0.3170188387650512141, 0.3333333333333333703, 0.3170188387650512141, 0.3333333333333333703, 0.3170188387650512141, 0.3333333333333333703, 0.3170188387650512141, 0.3333333333333333703, 0.3170188387650512141, 0.3333333333333333703, 0.3170188387650512141, 0.3333333333333333703, 0.3170188387650512141, 0.3333333333333333703, 0.3170188387650512141, 0.3333333333333333703, 0.3170188387650512141, 0.3333333333333333703, 0.3170188387650512141, 0.3333333333333333703, 0.3170188387650512141, 0.3333333333333333703, 0.3170188387650512141, 0.3333333333333333703, 0.3170188387650512141, 0.3333333333333333703, 0.3170188387650512141, 0.3333333333333333703, 0.3170188387650512141, 0.3333333333333333703, 0.3170188387650512141, 0.3333333333333333703, 0.3170188387650512141, 0.3333333333333333703, 0.3170188387650512141, 0.3333333333333333703, 0.3170188387650512141, 0.3333333333333333703, 0.3170188387650512141, 0.3333333333333333703, 0.3170188387650512141, 0.3333333333333333703, 0.3170188387650512141, 0.3333333333333333703, 0.3170188387650512141, 0.3333333333333333703, 0.3170188387650512141, 0.3333333333333333703, 0.3170188387650512141, 0.3333333333333333703, 0.3170188387650512141, 0.3333333333333333703, 0.3170188387650512141, 0.3333333333333333703, 0.3170188387650512141, 0.3333333333333333703, 0.3170188387650512141, 0.3333333333333333703, 0.3170188387650512141, 0.3333333333333333703, 0.3170188387650512141, 0.3333333333333333703, 0.3170188387650512141, 0.3333333333333333703, 0.3170188387650512141, 0.3333333333333333703, 0.3170188387650512141, 0.3333333333333333703, 0.3170188387650512141, 0.3333333333333333703, 0.3170188387650512141, 0.3333333333333333703, 0.3170188387650512141, 0.3333333333333333703, 0.3170188387650512141, 0.3333333333333333703, 0.3170188387650512141, 0.3333333333333333703, 0.3170188387650512141, 0.3333333333333333703, 0.3170188387650512141, 0.3333333333333333703, 0.3170188387650512141, 0.3333333333333333703, 0.3170188387650512141, 0.3333333333333333703, 0.3170188387650512141, 0.3333333333333333703, 0.3170188387650512141, 0.3333333333333333703, 0.3170188387650512141, 0.3333333333333333703, 0.3170188387650512141, 0.3333333333333333703, 0.3170188387650512141, 0.3333333333333333703, 0.3170188387650512141, 0.3333333333333333703, 0.3170188387650512141, 0.3333333333333333703, 0.3170188387650512141, 0.3333333333333333703, 0.3170188387650512141, 0.3333333333333333703, 0.3170188387650512141, 0.3333333333333333703, 0.3170188387650512141, 0.3333333333333333703, 0.3170188387650512141, 0.3333333333333333703, 0.3170188387650512141, 0.3333333333333333703, 0.3170188387650512141, 0.3333333333333333703, 0.3170188387650512141, 0.3333333333333333703, 0.3170188387650512141, 0.3333333333333333703, 0.3170188387650512141, 0.3333333333333333703, 0.3170188387650512141, 0.3333333333333333703, 0.3170188387650512141, 0.3333333333333333703, 0.3170188387650512141, 0.3333333333333333703, 0.3170188387650512141, 0.3333333333333333703, 0.3170188387650512141, 0.3333333333333333703, 0.3170188387650512141, 0.3333333333333333703, 0.3170188387650512141, 0.3333333333333333703),
 ( 0.3333333333333333703, 0.3170188387650512141, 0.3333333333333333703, 0.3170188387650512141, 0.3333333333333333703, 0.3170188387650512141, 0.3333333333333333703, 0.3170188387650512141, 0.3333333333333333703, 0.3170188387650512141, 0.3333333333333333703, 0.3170188387650512141, 0.3333333333333333703, 0.3170188387650512141, 0.3333333333333333703, 0.3170188387650512141, 0.3333333333333333703, 0.3170188387650512141, 0.3333333333333333703, 0.3170188387650512141, 0.3333333333333333703, 0.3170188387650512141, 0.3333333333333333703, 0.3170188387650512141, 0.3333333333333333703, 0.3170188387650512141, 0.3333333333333333703, 0.3170188387650512141, 0.3333333333333333703, 0.3170188387650512141, 0.3333333333333333703, 0.3170188387650512141, 0.3333333333333333703, 0.3170188387650512141, 0.3333333333333333703, 0.3170188387650512141, 0.3333333333333333703, 0.3170188387650512141, 0.3333333333333333703, 0.3170188387650512141, 0.3333333333333333703, 0.3170188387650512141, 0.3333333333333333703, 0.3170188387650512141, 0.3333333333333333703, 0.3170188387650512141, 0.3333333333333333703, 0.3170188387650512141, 0.3333333333333333703, 0.3170188387650512141, 0.3333333333333333703, 0.3170188387650512141, 0.3333333333333333703, 0.3170188387650512141, 0.3333333333333333703, 0.3170188387650512141, 0.3333333333333333703, 0.3170188387650512141, 0.3333333333333333703, 0.3170188387650512141, 0.3333333333333333703, 0.3170188387650512141, 0.3333333333333333703, 0.3170188387650512141, 0.3333333333333333703, 0.3170188387650512141, 0.3333333333333333703, 0.3170188387650512141, 0.3333333333333333703, 0.3170188387650512141, 0.3333333333333333703, 0.3170188387650512141, 0.3333333333333333703, 0.3170188387650512141, 0.3333333333333333703, 0.3170188387650512141, 0.3333333333333333703, 0.3170188387650512141, 0.3333333333333333703, 0.3170188387650512141, 0.3333333333333333703, 0.3170188387650512141, 0.3333333333333333703, 0.3170188387650512141, 0.3333333333333333703, 0.3170188387650512141, 0.3333333333333333703, 0.3170188387650512141, 0.3333333333333333703, 0.3170188387650512141, 0.3333333333333333703, 0.3170188387650512141, 0.3333333333333333703, 0.3170188387650512141, 0.3333333333333333703, 0.3170188387650512141, 0.3333333333333333703, 0.3170188387650512141, 0.3333333333333333703, 0.3170188387650512141, 0.3333333333333333703, 0.3170188387650512141, 0.3333333333333333703, 0.3170188387650512141, 0.3333333333333333703, 0.3170188387650512141, 0.3333333333333333703, 0.3170188387650512141, 0.3333333333333333703, 0.3170188387650512141, 0.3333333333333333703, 0.3170188387650512141, 0.3333333333333333703, 0.3170188387650512141, 0.3333333333333333703, 0.3170188387650512141, 0.3333333333333333703, 0.3170188387650512141, 0.3333333333333333703, 0.3170188387650512141, 0.3333333333333333703, 0.3170188387650512141, 0.3333333333333333703, 0.3170188387650512141, 0.3333333333333333703, 0.3170188387650512141, 0.3333333333333333703, 0.3170188387650512141, 0.3333333333333333703, 0.3170188387650512141, 0.3333333333333333703, 0.3170188387650512141, 0.3333333333333333703, 0.3170188387650512141, 0.3333333333333333703, 0.3170188387650512141, 0.3333333333333333703, 0.3170188387650512141, 0.3333333333333333703, 0.3170188387650512141, 0.3333333333333333703),
 ( 1.000000000000000000, 0.9510565162951535312, 1.000000000000000000, 0.9510565162951535312, 1.000000000000000000, 0.9510565162951535312, 1.000000000000000000, 0.9510565162951535312, 1.000000000000000000, 0.9510565162951535312, 1.000000000000000000, 0.9510565162951535312, 1.000000000000000000, 0.9510565162951535312, 1.000000000000000000, 0.9510565162951535312, 1.000000000000000000, 0.9510565162951535312, 1.000000000000000000, 0.9510565162951535312, 1.000000000000000000, 0.9510565162951535312, 1.000000000000000000, 0.9510565162951535312, 1.000000000000000000, 0.9510565162951535312, 1.000000000000000000, 0.9510565162951535312, 1.000000000000000000, 0.9510565162951535312, 1.000000000000000000, 0.9510565162951535312, 1.000000000000000000, 0.9510565162951535312, 1.000000000000000000, 0.9510565162951535312, 1.000000000000000000, 0.9510565162951535312, 1.000000000000000000, 0.9510565162951535312, 1.000000000000000000, 0.9510565162951535312, 1.000000000000000000, 0.9510565162951535312, 1.000000000000000000, 0.9510565162951535312, 1.000000000000000000, 0.9510565162951535312, 1.000000000000000000, 0.9510565162951535312, 1.000000000000000000, 0.9510565162951535312, 1.000000000000000000, 0.9510565162951535312, 1.000000000000000000, 0.9510565162951535312, 1.000000000000000000, 0.9510565162951535312, 1.000000000000000000, 0.9510565162951535312, 1.000000000000000000, 0.9510565162951535312, 1.000000000000000000, 0.9510565162951535312, 1.000000000000000000, 0.9510565162951535312, 1.000000000000000000, 0.9510565162951535312, 1.000000000000000000, 0.9510565162951535312, 1.000000000000000000, 0.9510565162951535312, 1.000000000000000000, 0.9510565162951535312, 1.000000000000000000, 0.9510565162951535312, 1.000000000000000000, 0.9510565162951535312, 1.000000000000000000, 0.9510565162951535312, 1.000000000000000000, 0.9510565162951535312, 1.000000000000000000, 0.9510565162951535312, 1.000000000000000000, 0.9510565162951535312, 1.000000000000000000, 0.9510565162951535312, 1.000000000000000000, 0.9510565162951535312, 1.000000000000000000, 0.9510565162951535312, 1.000000000000000000, 0.9510565162951535312, 1.000000000000000000, 0.9510565162951535312, 1.000000000000000000, 0.9510565162951535312, 1.000000000000000000, 0.9510565162951535312, 1.000000000000000000, 0.9510565162951535312, 1.000000000000000000, 0.9510565162951535312, 1.000000000000000000, 0.9510565162951535312, 1.000000000000000000, 0.9510565162951535312, 1.000000000000000000, 0.9510565162951535312, 1.000000000000000000, 0.9510565162951535312, 1.000000000000000000, 0.9510565162951535312, 1.000000000000000000, 0.9510565162951535312, 1.000000000000000000, 0.9510565162951535312, 1.000000000000000000, 0.9510565162951535312, 1.000000000000000000, 0.9510565162951535312, 1.000000000000000000, 0.9510565162951535312, 1.000000000000000000, 0.9510565162951535312, 1.000000000000000000, 0.9510565162951535312, 1.000000000000000000, 0.9510565162951535312, 1.000000000000000000, 0.9510565162951535312, 1.000000000000000000, 0.9510565162951535312, 1.000000000000000000, 0.9510565162951535312, 1.000000000000000000, 0.9510565162951535312, 1.000000000000000000, 0.9510565162951535312, 1.000000000000000000) ) ) 
 REPRESENTATION_ITEM ( '' )  SURFACE ( )  );
#5581=CARTESIAN_POINT ( 'NONE',  ( -31.38201786482021305, -40.29859572486944330, -8.387063443159975762 ) ) ;
#5582=CARTESIAN_POINT ( 'NONE',  ( -37.06321265474346660, -44.25000000000000000, 7.063212654743582952 ) ) ;
#5584=CARTESIAN_POINT ( 'NONE',  ( -28.51387258211773812, -49.80000000000001137, 9.383039235653802379 ) ) ;
#5594=CARTESIAN_POINT ( 'NONE',  ( -24.02705286092866643, -45.50140427513058228, 6.047868141099968398 ) ) ;
#5599=CARTESIAN_POINT ( 'NONE',  ( -36.01040764008574513, -48.00000000000000711, -6.010407640085605685 ) ) ;
#5603=CARTESIAN_POINT ( 'NONE',  ( -21.60464910494133406, -40.20000000000000995, 1.329692952841886155 ) ) ;
#5606=CARTESIAN_POINT ( 'NONE',  ( -34.53486167607238144, -30.15000000000000213, -8.900167166472096270 ) ) ;
#5610=CARTESIAN_POINT ( 'NONE',  ( -34.31290974752564438, -38.10000000000000853, 8.464561979789547053 ) ) ;
#5615=CARTESIAN_POINT ( 'NONE',  ( -21.59636165304264921, -35.19859572486944188, 1.277368040863740228 ) ) ;
#5616=CARTESIAN_POINT ( 'NONE',  ( -38.92545601287626056, -45.84859572486944046, -4.485229520447501450 ) ) ;
#5617=CARTESIAN_POINT ( 'NONE',  ( -31.27736804086391942, -29.30140427513058299, -8.403638346957361449 ) ) ;
#5627=CARTESIAN_POINT ( 'NONE',  ( -21.18131961722757595, -38.04859572486944330, -1.453139578080854699 ) ) ;
#5628=CARTESIAN_POINT ( 'NONE',  ( -39.86591130483550671, -44.55000000000001137, 1.562606840307984468 ) ) ;
#5630=CARTESIAN_POINT ( 'NONE',  ( -28.38237549136062654, -29.45140427513057801, -9.857197362228843573 ) ) ;
#5638=CARTESIAN_POINT ( 'NONE',  ( -22.03669253526174998, -34.35000000000000853, 4.057507815433014642 ) ) ;
#5648=CARTESIAN_POINT ( 'NONE',  ( -25.94249218456686279, -37.65000000000000568, 7.963307464738195840 ) ) ;
#5652=CARTESIAN_POINT ( 'NONE',  ( -31.48612741788231517, -36.30000000000000426, -9.383039235653804155 ) ) ;
#5654=CARTESIAN_POINT ( 'NONE',  ( -22.93678734525658314, -39.75000000000000000, -7.063212654743582064 ) ) ;
#5656=CARTESIAN_POINT ( 'NONE',  ( -36.01040764008574513, -51.00000000000000711, -6.010407640085605685 ) ) ;
#5658=CARTESIAN_POINT ( 'NONE',  ( -36.04786814110010340, -39.99859572486943904, -5.972947139071243861 ) ) ;
#5659=CARTESIAN_POINT ( 'NONE',  ( -34.26570676250101855, -51.09859572486944046, 8.488613101951703044 ) ) ;
#5661=CARTESIAN_POINT ( 'NONE',  ( -38.38706344316003793, -31.70140427513057091, -1.382017864820032083 ) ) ;
#5664=CARTESIAN_POINT ( 'NONE',  ( -28.51387258211773812, -31.80000000000000782, 9.383039235653802379 ) ) ;
#5671=CARTESIAN_POINT ( 'NONE',  ( -26.18828373723858149, -37.59859572486943335, -7.597606577763319713 ) ) ;
#5672=CARTESIAN_POINT ( 'NONE',  ( -34.53486167607238144, -42.15000000000001279, -8.900167166472096270 ) ) ;
#5675=CARTESIAN_POINT ( 'NONE',  ( -23.31994607974211675, -30.50140427513058583, 6.754974922286503869 ) ) ;
#5683=CARTESIAN_POINT ( 'NONE',  ( -21.60464910494133406, -34.20000000000000995, 1.329692952841886155 ) ) ;
#5693=CARTESIAN_POINT ( 'NONE',  ( -37.57355545560112375, -41.40000000000000568, 3.858919247786223305 ) ) ;
#5695=CARTESIAN_POINT ( 'NONE',  ( -23.68028341417693738, -30.75000000000000000, -6.319716585823200283 ) ) ;
#5696=CARTESIAN_POINT ( 'NONE',  ( -22.93678734525658314, -36.75000000000000711, -7.063212654743582952 ) ) ;
#5698=CARTESIAN_POINT ( 'NONE',  ( -36.71751442127229836, -39.00000000000000711, -6.717514421272142044 ) ) ;
#5701=CARTESIAN_POINT ( 'NONE',  ( -23.71967171589458445, -37.74859572486943904, -6.359104887540838469 ) ) ;
#5702=CARTESIAN_POINT ( 'NONE',  ( -31.48612741788231517, -30.30000000000000782, -9.383039235653804155 ) ) ;
#5703=CARTESIAN_POINT ( 'NONE',  ( -21.51138689804841420, -47.90140427513058086, -4.265706762501151772 ) ) ;
#5708=CARTESIAN_POINT ( 'NONE',  ( -39.38303923565386100, -32.70000000000000995, -1.486127417882099788 ) ) ;
#5716=CARTESIAN_POINT ( 'NONE',  ( -36.28032828410546529, -42.24859572486943904, 6.359104887540839357 ) ) ;
#5717=CARTESIAN_POINT ( 'NONE',  ( -25.68709025247441602, -42.60000000000000853, -8.464561979789547053 ) ) ;
#5719=CARTESIAN_POINT ( 'NONE',  ( -38.48861310195163554, -31.40140427513058086, 4.265706762501153548 ) ) ;
#5726=ORIENTED_EDGE ( 'NONE', *, *, #3403, .F. ) ;
#5728=CARTESIAN_POINT ( 'NONE',  ( -25.99212434019154472, -48.65140427513057375, 7.988596311142242890 ) ) ;
#5729=COLOUR_RGB ( '', 0.08235294, 0.09019608, 0.10196078) ;
#5738=CARTESIAN_POINT ( 'NONE',  ( -22.03669253526174998, -43.35000000000000853, 4.057507815433014642 ) ) ;
#5742=CARTESIAN_POINT ( 'NONE',  ( -25.46513832392765408, -34.64999999999998437, 8.900167166472096270 ) ) ;
#5745=CARTESIAN_POINT ( 'NONE',  ( -31.56260684030781505, -37.94999999999999574, 9.865911304835508489 ) ) ;
#5747=CARTESIAN_POINT ( 'NONE',  ( -34.58449383169706692, -31.14859572486944828, -8.874878320068054549 ) ) ;
#5748=CARTESIAN_POINT ( 'NONE',  ( -28.46154767013959486, -50.79859572486945041, 9.374751783755112200 ) ) ;
#5749=CARTESIAN_POINT ( 'NONE',  ( -21.61293655684001536, -30.20140427513057446, 1.382017864820032971 ) ) ;
#5752=CARTESIAN_POINT ( 'NONE',  ( -39.86591130483550671, -41.55000000000001137, 1.562606840307984468 ) ) ;
#5759=CARTESIAN_POINT ( 'NONE',  ( -38.40363834695740053, -45.69859572486943478, -1.277368040863739118 ) ) ;
#5760=CARTESIAN_POINT ( 'NONE',  ( -20.13408869516453947, -46.05000000000001137, -1.562606840307983136 ) ) ;
#5763=CARTESIAN_POINT ( 'NONE',  ( -28.38237549136062654, -35.45140427513057801, -9.857197362228843573 ) ) ;
#5770=APPLICATION_CONTEXT ( 'automotive_design' ) ;
#5771=CARTESIAN_POINT ( 'NONE',  ( -23.68028341417693738, -30.75000000000000000, -6.319716585823198507 ) ) ;
#5785=CARTESIAN_POINT ( 'NONE',  ( -37.06321265474346660, -38.25000000000000711, 7.063212654743582952 ) ) ;
#5788=CARTESIAN_POINT ( 'NONE',  ( -25.73429323749904185, -31.59859572486943335, -8.488613101951701267 ) ) ;
#5789=CARTESIAN_POINT ( 'NONE',  ( -31.56260684030781505, -40.95000000000000995, 9.865911304835510265 ) ) ;
#5790=CARTESIAN_POINT ( 'NONE',  ( -33.90612223281073057, -37.10140427513057659, 7.549504333439023718 ) ) ;
#5795=CARTESIAN_POINT ( 'NONE',  ( -22.93678734525658314, -36.75000000000000711, -7.063212654743582952 ) ) ;
#5803=CARTESIAN_POINT ( 'NONE',  ( -28.46154767013959486, -32.79859572486943620, 9.374751783755112200 ) ) ;
#5804=CARTESIAN_POINT ( 'NONE',  ( -23.28248557872775137, -49.50000000000000711, 6.717514421272141156 ) ) ;
#5807=CARTESIAN_POINT ( 'NONE',  ( -38.48861310195163554, -40.40140427513058086, 4.265706762501153548 ) ) ;
#5816=CARTESIAN_POINT ( 'NONE',  ( -22.06198138166579170, -48.35140427513057659, 4.107139971057695682 ) ) ;
#5829=CARTESIAN_POINT ( 'NONE',  ( -20.61696076434619584, -49.20000000000000995, 1.486127417882100676 ) ) ;
#5832=CARTESIAN_POINT ( 'NONE',  ( -22.97617564697422665, -31.74859572486943193, -7.102600956461224690 ) ) ;
#5833=CARTESIAN_POINT ( 'NONE',  ( -36.71751442127229836, -33.00000000000000711, -6.717514421272142044 ) ) ;
#5834=CARTESIAN_POINT ( 'NONE',  ( -36.35910488754074521, -40.25140427513058228, 6.280328284105565650 ) ) ;
#5837=CARTESIAN_POINT ( 'NONE',  ( -20.60867331244750034, -35.19859572486944188, 1.433802505903951419 ) ) ;
#5838=CARTESIAN_POINT ( 'NONE',  ( -28.51387258211773812, -37.80000000000000426, 9.383039235653802379 ) ) ;
#5839=FACE_OUTER_BOUND ( 'NONE', #3566, .T. ) ;
#5845=CARTESIAN_POINT ( 'NONE',  ( -28.65689575858256077, -46.44859572486943478, -8.836108267985801845 ) ) ;
#5846=CARTESIAN_POINT ( 'NONE',  ( -23.31994607974211675, -33.50140427513058228, 6.754974922286503869 ) ) ;
#5849=CARTESIAN_POINT ( 'NONE',  ( -21.51138689804841420, -32.90140427513058086, -4.265706762501151772 ) ) ;
#5857=CARTESIAN_POINT ( 'NONE',  ( -22.03669253526174998, -43.35000000000000853, 4.057507815433014642 ) ) ;
#5865=CARTESIAN_POINT ( 'NONE',  ( -22.40239342223677355, -35.90140427513058086, -3.811716262761597473 ) ) ;
#5868=CARTESIAN_POINT ( 'NONE',  ( -28.60187809025093841, -39.45000000000000284, -8.827394325379140483 ) ) ;
#5876=CARTESIAN_POINT ( 'NONE',  ( -36.28032828410546529, -48.24859572486943904, 6.359104887540839357 ) ) ;
#5877=CARTESIAN_POINT ( 'NONE',  ( -28.43739315969223824, -39.45000000000000995, -9.865911304835512041 ) ) ;
#5878=CARTESIAN_POINT ( 'NONE',  ( -24.02705286092866643, -39.50140427513058228, 6.047868141099968398 ) ) ;
#5883=CARTESIAN_POINT ( 'NONE',  ( -20.60867331244750034, -41.19859572486944188, 1.433802505903951419 ) ) ;
#5884=CARTESIAN_POINT ( 'NONE',  ( -20.61696076434619584, -40.20000000000000995, 1.486127417882100676 ) ) ;
#5892=CARTESIAN_POINT ( 'NONE',  ( -34.58449383169706692, -34.14859572486943051, -8.874878320068054549 ) ) ;
#5893=CARTESIAN_POINT ( 'NONE',  ( -36.71751442127229836, -51.00000000000000711, -6.717514421272142044 ) ) ;
#5896=CARTESIAN_POINT ( 'NONE',  ( -22.89739904353894318, -38.75140427513058228, -7.023824353025938549 ) ) ;
#5902=CARTESIAN_POINT ( 'NONE',  ( -21.60464910494133406, -43.20000000000000995, 1.329692952841886155 ) ) ;
#5903=MANIFOLD_SOLID_BREP ( 'Sweep1', #2106 ) ;
#5907=CARTESIAN_POINT ( 'NONE',  ( -20.13408869516453947, -31.05000000000000782, -1.562606840307983136 ) ) ;
#5909=CARTESIAN_POINT ( 'NONE',  ( -37.93801861833426159, -31.85140427513056594, -4.107139971057695682 ) ) ;
#5912=CARTESIAN_POINT ( 'NONE',  ( -25.94249218456686279, -34.64999999999999858, 7.963307464738194952 ) ) ;
#5917=CARTESIAN_POINT ( 'NONE',  ( -33.81171626276147890, -45.09859572486944046, 7.597606577763319713 ) ) ;
#5918=CARTESIAN_POINT ( 'NONE',  ( -34.53486167607238144, -33.15000000000001279, -8.900167166472096270 ) ) ;
#5919=CARTESIAN_POINT ( 'NONE',  ( -37.93801861833426159, -37.85140427513057659, -4.107139971057695682 ) ) ;
#5923=CARTESIAN_POINT ( 'NONE',  ( -21.07454398712378918, -38.34859572486944046, 4.485229520447505003 ) ) ;
#5924=CARTESIAN_POINT ( 'NONE',  ( -23.28248557872775137, -43.50000000000001421, 6.717514421272141156 ) ) ;
#5930=CARTESIAN_POINT ( 'NONE',  ( -21.59636165304264921, -50.19859572486944188, 1.277368040863740228 ) ) ;
#5931=CARTESIAN_POINT ( 'NONE',  ( -31.43380250590416125, -35.30140427513057944, -9.391326687552492558 ) ) ;
#5934=CARTESIAN_POINT ( 'NONE',  ( -36.68005392025794009, -47.00140427513058938, -6.754974922286504757 ) ) ;
#5941=CARTESIAN_POINT ( 'NONE',  ( -23.68028341417693738, -39.74999999999999289, -6.319716585823198507 ) ) ;
#5947=CARTESIAN_POINT ( 'NONE',  ( -25.46513832392765408, -40.65000000000000568, 8.900167166472096270 ) ) ;
#5951=CARTESIAN_POINT ( 'NONE',  ( -31.27736804086391942, -38.30140427513057944, -8.403638346957361449 ) ) ;
#5954=CARTESIAN_POINT ( 'NONE',  ( -21.60464910494133406, -40.20000000000000995, 1.329692952841886155 ) ) ;
#5956=CARTESIAN_POINT ( 'NONE',  ( -22.93678734525658314, -45.75000000000000000, -7.063212654743582064 ) ) ;
#5960=CARTESIAN_POINT ( 'NONE',  ( -39.38303923565386100, -32.70000000000000995, -1.486127417882099788 ) ) ;
#5961=CARTESIAN_POINT ( 'NONE',  ( -38.83610826798580717, -46.55140427513058654, 1.343104241417631073 ) ) ;
#5965=CARTESIAN_POINT ( 'NONE',  ( -39.85719736222883824, -33.54859572486944330, 1.617624508639602388 ) ) ;
#5971=CARTESIAN_POINT ( 'NONE',  ( -34.05750781543318340, -45.14999999999999858, -7.963307464738195840 ) ) ;
#5973=CARTESIAN_POINT ( 'NONE',  ( -37.02382435302582309, -33.24859572486943193, 7.102600956461226467 ) ) ;
#5974=CARTESIAN_POINT ( 'NONE',  ( -38.48861310195163554, -31.40140427513058086, 4.265706762501153548 ) ) ;
#5976=CARTESIAN_POINT ( 'NONE',  ( -25.63988726744978663, -47.60140427513058370, -8.440510857627391061 ) ) ;
#5983=CARTESIAN_POINT ( 'NONE',  ( -23.68028341417693738, -45.74999999999999289, -6.319716585823198507 ) ) ;
#5989=CARTESIAN_POINT ( 'NONE',  ( -21.09983283352784156, -46.34999999999998721, 4.534861676072186043 ) ) ;
#5992=CARTESIAN_POINT ( 'NONE',  ( -34.00787565980851213, -38.15140427513058086, -7.988596311142238449 ) ) ;
#5994=CARTESIAN_POINT ( 'NONE',  ( -34.05750781543319050, -33.15000000000000568, -7.963307464738194952 ) ) ;
#6001=CARTESIAN_POINT ( 'NONE',  ( -31.48612741788231517, -45.30000000000000426, -9.383039235653804155 ) ) ;
#6002=CARTESIAN_POINT ( 'NONE',  ( -21.61293655684001536, -48.20140427513058512, 1.382017864820032971 ) ) ;
#6007=CARTESIAN_POINT ( 'NONE',  ( -38.44051085762733777, -36.39859572486944472, 4.360112732550414982 ) ) ;
#6015=CARTESIAN_POINT ( 'NONE',  ( -38.82739432537914581, -50.55000000000001137, 1.398121909749243441 ) ) ;
#6016=CARTESIAN_POINT ( 'NONE',  ( -20.60867331244750034, -41.19859572486944188, 1.433802505903951419 ) ) ;
#6017=CARTESIAN_POINT ( 'NONE',  ( -22.89739904353894318, -44.75140427513058228, -7.023824353025938549 ) ) ;
#6019=ORIENTED_EDGE ( 'NONE', *, *, #6970, .F. ) ;
#6020=CARTESIAN_POINT ( 'NONE',  ( -28.56619749409589204, -48.80140427513057233, 9.391326687552490782 ) ) ;
#6028=CARTESIAN_POINT ( 'NONE',  ( -37.57355545560112375, -44.40000000000000568, 3.858919247786223305 ) ) ;
#6029=CARTESIAN_POINT ( 'NONE',  ( -38.90016716647221529, -35.84999999999998721, -4.534861676072185155 ) ) ;
#6033=CARTESIAN_POINT ( 'NONE',  ( -31.56260684030781505, -40.95000000000000995, 9.865911304835510265 ) ) ;
#6035=CARTESIAN_POINT ( 'NONE',  ( -25.99212434019154472, -33.65140427513057375, 7.988596311142242890 ) ) ;
#6038=CARTESIAN_POINT ( 'NONE',  ( -23.68028341417693738, -39.75000000000000000, -6.319716585823200283 ) ) ;
#6044=CARTESIAN_POINT ( 'NONE',  ( -22.93678734525658314, -42.75000000000001421, -7.063212654743582952 ) ) ;
#6045=CARTESIAN_POINT ( 'NONE',  ( -21.16389173201424612, -48.05140427513057233, -1.343104241417630185 ) ) ;
#6049=CARTESIAN_POINT ( 'NONE',  ( -28.46154767013959486, -47.79859572486944330, 9.374751783755112200 ) ) ;
#6057=CARTESIAN_POINT ( 'NONE',  ( -22.01140368885771892, -32.34859572486942625, 4.007875659808335378 ) ) ;
#6058=CARTESIAN_POINT ( 'NONE',  ( -34.26570676250101855, -39.09859572486944046, 8.488613101951703044 ) ) ;
#6059=CARTESIAN_POINT ( 'NONE',  ( -20.12537475255788522, -45.05140427513057944, -1.507589171976365439 ) ) ;
#6064=CARTESIAN_POINT ( 'NONE',  ( -38.87487832006816291, -46.85140427513056949, -4.584493831696867971 ) ) ;
#6071=CARTESIAN_POINT ( 'NONE',  ( -37.57355545560112375, -47.40000000000001279, 3.858919247786223305 ) ) ;
#6073=CARTESIAN_POINT ( 'NONE',  ( -21.09983283352784156, -34.35000000000000853, 4.534861676072186043 ) ) ;
#6074=PRODUCT_DEFINITION_FORMATION_WITH_SPECIFIED_SOURCE ( 'ANY', '', #3813, .NOT_KNOWN. ) ;
#6078=CARTESIAN_POINT ( 'NONE',  ( -38.90016716647221529, -44.85000000000001563, -4.534861676072185155 ) ) ;
#6081=CARTESIAN_POINT ( 'NONE',  ( -34.00787565980851213, -41.15140427513058086, -7.988596311142238449 ) ) ;
#6085=( GEOMETRIC_REPRESENTATION_CONTEXT ( 3 ) GLOBAL_UNCERTAINTY_ASSIGNED_CONTEXT ( ( #5459 ) ) GLOBAL_UNIT_ASSIGNED_CONTEXT ( ( #974, #841, #1591 ) ) REPRESENTATION_CONTEXT ( 'NONE', 'WORKASPACE' ) );
#6086=CARTESIAN_POINT ( 'NONE',  ( -28.60187809025093841, -48.45000000000000284, -8.827394325379140483 ) ) ;
#6092=CARTESIAN_POINT ( 'NONE',  ( -34.53486167607238144, -48.15000000000001279, -8.900167166472096270 ) ) ;
#6093=CARTESIAN_POINT ( 'NONE',  ( -28.60187809025093841, -30.44999999999999574, -8.827394325379140483 ) ) ;
#6096=CARTESIAN_POINT ( 'NONE',  ( -20.60867331244750034, -44.19859572486944899, 1.433802505903951419 ) ) ;
#6101=CARTESIAN_POINT ( 'NONE',  ( -28.60187809025093841, -48.44999999999999574, -8.827394325379140483 ) ) ;
#6102=CARTESIAN_POINT ( 'NONE',  ( -28.49241082802385350, -40.44859572486944188, -9.874625247442173404 ) ) ;
#6103=CARTESIAN_POINT ( 'NONE',  ( -28.56619749409589204, -45.80140427513057944, 9.391326687552490782 ) ) ;
#6108=CARTESIAN_POINT ( 'NONE',  ( -36.68005392025794009, -44.00140427513057517, -6.754974922286504757 ) ) ;
#6117=CARTESIAN_POINT ( 'NONE',  ( -28.60187809025093841, -48.44999999999999574, -8.827394325379140483 ) ) ;
#6118=CARTESIAN_POINT ( 'NONE',  ( -38.90016716647221529, -38.85000000000001563, -4.534861676072185155 ) ) ;
#6126=CARTESIAN_POINT ( 'NONE',  ( -38.83610826798580717, -43.55140427513057944, 1.343104241417631073 ) ) ;
#6130=CARTESIAN_POINT ( 'NONE',  ( -28.67030704715798350, -49.80000000000001137, 8.395350895058669494 ) ) ;
#6137=CARTESIAN_POINT ( 'NONE',  ( -37.06321265474346660, -44.25000000000000000, 7.063212654743582952 ) ) ;
#6138=CARTESIAN_POINT ( 'NONE',  ( -36.01040764008574513, -33.00000000000000711, -6.010407640085605685 ) ) ;
#6144=CARTESIAN_POINT ( 'NONE',  ( -37.02382435302582309, -48.24859572486943904, 7.102600956461226467 ) ) ;
#6146=CARTESIAN_POINT ( 'NONE',  ( -20.13408869516454303, -34.04999999999999005, -1.562606840307982692 ) ) ;
#6149=DIRECTION ( 'NONE',  ( -0.7061138087190598212, 0.05297714858780487590, 0.7061138087190823587 ) ) ;
#6151=CARTESIAN_POINT ( 'NONE',  ( -37.96330746473829976, -47.85000000000000853, -4.057507815433013754 ) ) ;
#6152=CARTESIAN_POINT ( 'NONE',  ( -34.58449383169706692, -43.14859572486943762, -8.874878320068054549 ) ) ;
#6153=CARTESIAN_POINT ( 'NONE',  ( -38.87487832006816291, -40.85140427513057659, -4.584493831696867971 ) ) ;
#6165=CARTESIAN_POINT ( 'NONE',  ( -31.38201786482021305, -31.29859572486943975, -8.387063443159975762 ) ) ;
#6166=CARTESIAN_POINT ( 'NONE',  ( -20.13408869516453947, -31.05000000000000782, -1.562606840307983136 ) ) ;
#6168=CARTESIAN_POINT ( 'NONE',  ( -28.43739315969223824, -48.44999999999999574, -9.865911304835512041 ) ) ;
#6174=CARTESIAN_POINT ( 'NONE',  ( -21.61293655684001536, -39.20140427513058512, 1.382017864820032971 ) ) ;
#6176=CARTESIAN_POINT ( 'NONE',  ( -38.39535089505872634, -47.70000000000000284, -1.329692952841885267 ) ) ;
#6181=CARTESIAN_POINT ( 'NONE',  ( -36.71751442127229836, -51.00000000000000711, -6.717514421272142044 ) ) ;
#6182=CARTESIAN_POINT ( 'NONE',  ( -28.67030704715798350, -40.80000000000000426, 8.395350895058669494 ) ) ;
#6185=CARTESIAN_POINT ( 'NONE',  ( -31.53845232986046554, -43.29859572486943620, -9.374751783755117529 ) ) ;
#6186=DIRECTION ( 'NONE',  ( -0.7061138087190598212, 0.05297714858780487590, 0.7061138087190823587 ) ) ;
#6187=CARTESIAN_POINT ( 'NONE',  ( -31.48612741788231517, -30.30000000000000782, -9.383039235653804155 ) ) ;
#6191=CARTESIAN_POINT ( 'NONE',  ( -21.18131961722757595, -38.04859572486944330, -1.453139578080854699 ) ) ;
#6192=CARTESIAN_POINT ( 'NONE',  ( -31.50758917197619979, -38.94859572486943478, 9.874625247442176956 ) ) ;
#6193=CARTESIAN_POINT ( 'NONE',  ( -38.48861310195163554, -37.40140427513058796, 4.265706762501153548 ) ) ;
#6195=( BOUNDED_SURFACE ( )  B_SPLINE_SURFACE ( 3, 2, ( 
 ( #8281, #1478, #6854, #4881, #2242, #4964, #4921, #7518, #2989, #7601, #115, #1564, #5664, #8367, #2330, #1162, #1875, #6494, #5708, #1752, #8528, #7078, #4434, #7159, #6367, #3164, #367, #404, #8488, #4391, #6536, #3812, #5175, #8571, #3117, #1119, #485, #8451, #7117, #1079, #3035, #3773, #445, #1791, #6452, #5795, #7868, #3076, #7243, #2453, #5134, #7201, #5838, #2494, #3730, #4560, #7826, #4473, #8410, #1037, #1204, #3857, #2535, #1832, #4514, #5214, #3201, #6411, #5884, #329, #2375, #7909, #5050, #7740, #1702, #7781, #5092, #5752, #2414, #7952, #7286, #1915, #5254, #8615, #3242, #4603, #3899, #6577, #531, #2584, #5924, #1530, #4359, #4271, #6334, #7039, #1668, #917, #3528, #3001, #211, #5495, #7614, #4313, #8379, #8248, #869, #124, #3572, #2823, #6256, #6206, #1487, #3487, #2914, #6908, #2165, #3612, #4224, #8205, #2870, #7659, #828, #6168, #170, #4850, #5542, #1621, #2207, #7528, #4892, #6995, #5584, #4183, #8291, #6864, #7569, #2251, #4930, #6292, #1577 ),
 ( #6953, #254, #2956, #5630, #8330, #2296, #4978, #960, #3655, #298, #5675, #2338, #5019, #7709, #4444, #1714, #5719, #2547, #7169, #7879, #378, #7795, #4572, #4401, #5144, #6421, #5849, #4527, #7836, #8421, #3085, #1129, #5223, #3824, #7089, #6504, #4483, #7127, #8460, #1762, #1047, #3739, #5185, #5763, #1090, #2423, #457, #7213, #1803, #8581, #3172, #3212, #2385, #3785, #8540, #2508, #3870, #1175, #2463, #7922, #1000, #1846, #6546, #5104, #499, #5896, #3698, #6462, #1888, #415, #6378, #338, #3045, #5059, #3128, #7749, #5807, #8501, #1216, #3432, #7433, #5394, #3302, #4746, #2060, #66, #7389, #588, #1390, #3912, #1967, #8052, #1343, #1298, #3253, #4085, #6763, #2015, #2109, #726, #6108, #2770, #6588, #543, #4614, #3998, #5438, #682, #7964, #2637, #4704, #7254, #4042, #1255, #6678, #635, #5264, #8150, #6723, #6064, #5934, #3343, #3387, #8628, #5976, #5309, #8011, #2595, #4656, #23, #2681, #7343, #6020, #2724, #3953, #1928, #8709, #5350, #8103, #7298, #6630 ),
 ( #8669, #3883, #2656, #8072, #2520, #1902, #4629, #3318, #4015, #4673, #2610, #3139, #1143, #5278, #7314, #8598, #7983, #1986, #3837, #5909, #7362, #516, #2033, #4720, #1944, #652, #2563, #5326, #7227, #6518, #470, #6035, #1315, #8026, #5241, #6694, #3362, #2698, #1270, #3227, #5367, #3184, #4587, #3970, #6649, #3929, #5865, #8556, #5196, #604, #7892, #1859, #4541, #1188, #6563, #7935, #7271, #6603, #1231, #559, #3270, #5992, #5951, #8644, #8683, #4061, #1407, #6213, #6174, #6739, #2128, #2790, #1456, #84, #5549, #2214, #5456, #3404, #791, #219, #698, #6081, #4190, #40, #6871, #2170, #6827, #4857, #8212, #745, #7533, #2922, #1493, #8121, #833, #3535, #4809, #6126, #8166, #7451, #4103, #2877, #4766, #7493, #4149, #178, #4899, #1360, #6781, #8255, #5594, #2743, #3493, #7577, #1538, #4232, #6915, #131, #6263, #7406, #2829, #877, #5503, #3580, #8298, #5411, #3449, #2259, #2078, #5816, #8508, #5728, #4451, #968, #386, #2303, #7619, #1584, #1099, #5110, #3092 ),
 ( #4985, #7135, #1676, #6960, #345, #5771, #3792, #3663, #2346, #4278, #5027, #924, #7717, #7667, #2965, #4938, #4366, #8386, #3620, #5068, #3008, #6302, #4322, #8469, #1629, #3137, #7005, #2431, #5683, #5638, #7050, #261, #8338, #6344, #306, #7758, #1010, #3706, #1722, #6386, #6469, #3053, #8428, #7803, #2392, #1770, #422, #4409, #7096, #1054, #3747, #6431, #6554, #3261, #2471, #7974, #5191, #5231, #4580, #464, #2647, #8636, #1261, #4663, #7928, #5941, #5316, #4536, #507, #3220, #7843, #7177, #7261, #4006, #1810, #1138, #1936, #3832, #4621, #2603, #1895, #5271, #7306, #3179, #4492, #3877, #1223, #6595, #5902, #5857, #6512, #6685, #3961, #596, #1853, #8588, #6028, #8548, #551, #7887, #6638, #2555, #2516, #3920, #3310, #5983, #8676, #8017, #1976, #7220, #3352, #7351, #1306, #643, #5154, #1184, #6071, #6904, #5445, #6770, #5358, #6731, #8245, #6117, #2204, #5492, #1445, #7566, #3525, #30, #4179, #3567, #4713, #8157, #121, #1351, #4799, #1398, #7440, #734, #866 ),
 ( #4094, #6203, #6165, #4138, #1527, #5401, #4221, #3440, #8339, #780, #2865, #2689, #8059, #2820, #2731, #4889, #2116, #2023, #6818, #825, #7396, #4755, #72, #4051, #2780, #690, #7481, #8110, #3396, #2069, #3483, #8202, #2160, #4846, #7525, #1484, #6861, #167, #5539, #4441, #2953, #1043, #4309, #6948, #5671, #7610, #1571, #5627, #913, #334, #8327, #4927, #3041, #8457, #1664, #2420, #6417, #8373, #2911, #251, #5056, #5016, #5581, #956, #1618, #294, #7655, #4397, #3736, #6992, #2248, #2335, #7790, #8288, #4266, #5716, #3608, #8417, #996, #7705, #3694, #7036, #6289, #2291, #3652, #4356, #6374, #6330, #4972, #2996, #1758, #2381, #7086, #7746, #1710, #1085, #374, #3082, #5759, #5100, #7124, #6252, #208, #5845, #3906, #5303, #6584, #4480, #539, #7249, #7208, #2503, #4522, #3819, #6499, #7959, #1126, #1169, #5181, #3250, #1251, #6459, #452, #5260, #1963, #5141, #3864, #1211, #5930, #6625, #7294, #5220, #2632, #3782, #7918, #8623, #7875, #1882, #4609, #411, #8536 ),
 ( #1841, #3949, #2591, #4567, #8006, #3169, #4651, #6542, #7338, #1921, #583, #3123, #5803, #3299, #493, #5973, #3207, #8497, #8665, #2459, #7833, #5892, #8577, #1798, #2543, #7166, #1385, #1339, #8048, #1294, #6757, #4742, #8704, #1430, #8098, #7469, #5434, #2852, #6718, #5528, #2056, #2191, #2104, #4168, #4877, #8232, #4126, #4038, #814, #720, #3338, #8144, #2148, #6192, #6058, #7428, #6674, #4081, #630, #3428, #677, #2010, #3994, #6102, #62, #2676, #6807, #2766, #6016, #3382, #5479, #7385, #5345, #18, #4834, #4786, #4700, #768, #2719, #5389, #3471, #6152, #110, #2808, #8188, #7513, #1474, #6849, #3515, #155, #5045, #901, #2369, #3071, #7691, #6892, #2941, #985, #8274, #5616, #8362, #7554, #4344, #1561, #1606, #944, #5567, #7735, #5003, #6362, #1033, #4296, #2238, #1517, #1697, #8317, #2280, #4210, #4961, #2325, #2985, #7643, #6980, #325, #4255, #8446, #3640, #6321, #8405, #1652, #3683, #4917, #5748, #284, #5659, #855, #7597, #7073, #7024, #3725, #3031 ),
 ( #2408, #3554, #5702, #4387, #198, #6407, #238, #6279, #362, #6238, #2900, #6938, #3599, #4553, #5170, #3806, #2578, #1786, #5960, #1827, #5833, #5918, #2530, #7237, #2449, #3282, #4508, #3158, #1747, #3109, #4597, #2488, #7281, #1869, #6531, #3936, #8608, #5130, #525, #8654, #1074, #7195, #5207, #6448, #1154, #6488, #438, #8522, #5087, #3893, #7776, #1197, #6572, #7862, #3849, #5249, #7903, #479, #6614, #4468, #569, #3194, #4430, #5877, #7946, #7112, #3767, #3236, #7821, #1240, #8566, #400, #1909, #5789, #8483, #1114, #7153, #7994, #6, #1952, #2707, #2665, #616, #2619, #8084, #6044, #1280, #2754, #664, #4637, #1996, #6792, #8692, #802, #8036, #6137, #3370, #3327, #2042, #3980, #6660, #4686, #6001, #5421, #7371, #5333, #8131, #1325, #4157, #4730, #3414, #97, #4026, #2796, #6835, #2091, #7325, #6703, #4774, #5376, #7415, #6092, #5288, #7459, #1373, #4070, #6746, #709, #5465, #50, #1417, #4817, #4113, #756, #3459, #8174, #2137, #7501, #1462, #3503, #6181 ) ),
 .UNSPECIFIED., .T., .F., .T. ) 
 B_SPLINE_SURFACE_WITH_KNOTS ( ( 4, 3, 4 ),
 ( 3, 2, 2, 2, 2, 2, 2, 2, 2, 2, 2, 2, 2, 2, 2, 2, 2, 2, 2, 2, 2, 2, 2, 2, 2, 2, 2, 2, 2, 2, 2, 2, 2, 2, 2, 2, 2, 2, 2, 2, 2, 2, 2, 2, 2, 2, 2, 2, 2, 2, 2, 2, 2, 2, 2, 2, 2, 2, 2, 2, 2, 2, 2, 2, 2, 2, 2, 2, 2, 2, 3 ),
 ( 0.000000000000000000, 0.5000000000000000000, 1.000000000000000000 ),
 ( 0.000000000000000000, 0.01428571428571428527, 0.02857142857142857054, 0.04285714285714285754, 0.05714285714285714107, 0.07142857142857142461, 0.08571428571428571508, 0.1000000000000000056, 0.1142857142857142821, 0.1285714285714285587, 0.1428571428571428492, 0.1571428571428571397, 0.1714285714285714302, 0.1857142857142857206, 0.2000000000000000111, 0.2142857142857142738, 0.2285714285714285643, 0.2428571428571428548, 0.2571428571428571175, 0.2714285714285714080, 0.2857142857142856984, 0.2999999999999999889, 0.3142857142857142794, 0.3285714285714285698, 0.3428571428571428603, 0.3571428571428571508, 0.3714285714285714413, 0.3857142857142857317, 0.4000000000000000222, 0.4142857142857143127, 0.4285714285714285476, 0.4428571428571428381, 0.4571428571428571286, 0.4714285714285714191, 0.4857142857142857095, 0.5000000000000000000, 0.5142857142857142350, 0.5285714285714285809, 0.5428571428571428159, 0.5571428571428571619, 0.5714285714285713969, 0.5857142857142857428, 0.5999999999999999778, 0.6142857142857143238, 0.6285714285714285587, 0.6428571428571429047, 0.6571428571428571397, 0.6714285714285713746, 0.6857142857142857206, 0.6999999999999999556, 0.7142857142857143016, 0.7285714285714285365, 0.7428571428571428825, 0.7571428571428571175, 0.7714285714285714635, 0.7857142857142856984, 0.8000000000000000444, 0.8142857142857142794, 0.8285714285714286254, 0.8428571428571428603, 0.8571428571428570953, 0.8714285714285714413, 0.8857142857142856762, 0.9000000000000000222, 0.9142857142857142572, 0.9285714285714286031, 0.9428571428571428381, 0.9571428571428571841, 0.9714285714285714191, 0.9857142857142857650, 1.000000000000000000 ),
 .UNSPECIFIED. ) 
 GEOMETRIC_REPRESENTATION_ITEM ( )  RATIONAL_B_SPLINE_SURFACE ( (
 ( 1.000000000000000000, 0.9510565162951535312, 1.000000000000000000, 0.9510565162951535312, 1.000000000000000000, 0.9510565162951535312, 1.000000000000000000, 0.9510565162951535312, 1.000000000000000000, 0.9510565162951535312, 1.000000000000000000, 0.9510565162951535312, 1.000000000000000000, 0.9510565162951535312, 1.000000000000000000, 0.9510565162951535312, 1.000000000000000000, 0.9510565162951535312, 1.000000000000000000, 0.9510565162951535312, 1.000000000000000000, 0.9510565162951535312, 1.000000000000000000, 0.9510565162951535312, 1.000000000000000000, 0.9510565162951535312, 1.000000000000000000, 0.9510565162951535312, 1.000000000000000000, 0.9510565162951535312, 1.000000000000000000, 0.9510565162951535312, 1.000000000000000000, 0.9510565162951535312, 1.000000000000000000, 0.9510565162951535312, 1.000000000000000000, 0.9510565162951535312, 1.000000000000000000, 0.9510565162951535312, 1.000000000000000000, 0.9510565162951535312, 1.000000000000000000, 0.9510565162951535312, 1.000000000000000000, 0.9510565162951535312, 1.000000000000000000, 0.9510565162951535312, 1.000000000000000000, 0.9510565162951535312, 1.000000000000000000, 0.9510565162951535312, 1.000000000000000000, 0.9510565162951535312, 1.000000000000000000, 0.9510565162951535312, 1.000000000000000000, 0.9510565162951535312, 1.000000000000000000, 0.9510565162951535312, 1.000000000000000000, 0.9510565162951535312, 1.000000000000000000, 0.9510565162951535312, 1.000000000000000000, 0.9510565162951535312, 1.000000000000000000, 0.9510565162951535312, 1.000000000000000000, 0.9510565162951535312, 1.000000000000000000, 0.9510565162951535312, 1.000000000000000000, 0.9510565162951535312, 1.000000000000000000, 0.9510565162951535312, 1.000000000000000000, 0.9510565162951535312, 1.000000000000000000, 0.9510565162951535312, 1.000000000000000000, 0.9510565162951535312, 1.000000000000000000, 0.9510565162951535312, 1.000000000000000000, 0.9510565162951535312, 1.000000000000000000, 0.9510565162951535312, 1.000000000000000000, 0.9510565162951535312, 1.000000000000000000, 0.9510565162951535312, 1.000000000000000000, 0.9510565162951535312, 1.000000000000000000, 0.9510565162951535312, 1.000000000000000000, 0.9510565162951535312, 1.000000000000000000, 0.9510565162951535312, 1.000000000000000000, 0.9510565162951535312, 1.000000000000000000, 0.9510565162951535312, 1.000000000000000000, 0.9510565162951535312, 1.000000000000000000, 0.9510565162951535312, 1.000000000000000000, 0.9510565162951535312, 1.000000000000000000, 0.9510565162951535312, 1.000000000000000000, 0.9510565162951535312, 1.000000000000000000, 0.9510565162951535312, 1.000000000000000000, 0.9510565162951535312, 1.000000000000000000, 0.9510565162951535312, 1.000000000000000000, 0.9510565162951535312, 1.000000000000000000, 0.9510565162951535312, 1.000000000000000000, 0.9510565162951535312, 1.000000000000000000, 0.9510565162951535312, 1.000000000000000000, 0.9510565162951535312, 1.000000000000000000, 0.9510565162951535312, 1.000000000000000000, 0.9510565162951535312, 1.000000000000000000, 0.9510565162951535312, 1.000000000000000000, 0.9510565162951535312, 1.000000000000000000, 0.9510565162951535312, 1.000000000000000000),
 ( 0.3333333333333333703, 0.3170188387650512141, 0.3333333333333333703, 0.3170188387650512141, 0.3333333333333333703, 0.3170188387650512141, 0.3333333333333333703, 0.3170188387650512141, 0.3333333333333333703, 0.3170188387650512141, 0.3333333333333333703, 0.3170188387650512141, 0.3333333333333333703, 0.3170188387650512141, 0.3333333333333333703, 0.3170188387650512141, 0.3333333333333333703, 0.3170188387650512141, 0.3333333333333333703, 0.3170188387650512141, 0.3333333333333333703, 0.3170188387650512141, 0.3333333333333333703, 0.3170188387650512141, 0.3333333333333333703, 0.3170188387650512141, 0.3333333333333333703, 0.3170188387650512141, 0.3333333333333333703, 0.3170188387650512141, 0.3333333333333333703, 0.3170188387650512141, 0.3333333333333333703, 0.3170188387650512141, 0.3333333333333333703, 0.3170188387650512141, 0.3333333333333333703, 0.3170188387650512141, 0.3333333333333333703, 0.3170188387650512141, 0.3333333333333333703, 0.3170188387650512141, 0.3333333333333333703, 0.3170188387650512141, 0.3333333333333333703, 0.3170188387650512141, 0.3333333333333333703, 0.3170188387650512141, 0.3333333333333333703, 0.3170188387650512141, 0.3333333333333333703, 0.3170188387650512141, 0.3333333333333333703, 0.3170188387650512141, 0.3333333333333333703, 0.3170188387650512141, 0.3333333333333333703, 0.3170188387650512141, 0.3333333333333333703, 0.3170188387650512141, 0.3333333333333333703, 0.3170188387650512141, 0.3333333333333333703, 0.3170188387650512141, 0.3333333333333333703, 0.3170188387650512141, 0.3333333333333333703, 0.3170188387650512141, 0.3333333333333333703, 0.3170188387650512141, 0.3333333333333333703, 0.3170188387650512141, 0.3333333333333333703, 0.3170188387650512141, 0.3333333333333333703, 0.3170188387650512141, 0.3333333333333333703, 0.3170188387650512141, 0.3333333333333333703, 0.3170188387650512141, 0.3333333333333333703, 0.3170188387650512141, 0.3333333333333333703, 0.3170188387650512141, 0.3333333333333333703, 0.3170188387650512141, 0.3333333333333333703, 0.3170188387650512141, 0.3333333333333333703, 0.3170188387650512141, 0.3333333333333333703, 0.3170188387650512141, 0.3333333333333333703, 0.3170188387650512141, 0.3333333333333333703, 0.3170188387650512141, 0.3333333333333333703, 0.3170188387650512141, 0.3333333333333333703, 0.3170188387650512141, 0.3333333333333333703, 0.3170188387650512141, 0.3333333333333333703, 0.3170188387650512141, 0.3333333333333333703, 0.3170188387650512141, 0.3333333333333333703, 0.3170188387650512141, 0.3333333333333333703, 0.3170188387650512141, 0.3333333333333333703, 0.3170188387650512141, 0.3333333333333333703, 0.3170188387650512141, 0.3333333333333333703, 0.3170188387650512141, 0.3333333333333333703, 0.3170188387650512141, 0.3333333333333333703, 0.3170188387650512141, 0.3333333333333333703, 0.3170188387650512141, 0.3333333333333333703, 0.3170188387650512141, 0.3333333333333333703, 0.3170188387650512141, 0.3333333333333333703, 0.3170188387650512141, 0.3333333333333333703, 0.3170188387650512141, 0.3333333333333333703, 0.3170188387650512141, 0.3333333333333333703, 0.3170188387650512141, 0.3333333333333333703, 0.3170188387650512141, 0.3333333333333333703, 0.3170188387650512141, 0.3333333333333333703, 0.3170188387650512141, 0.3333333333333333703),
 ( 0.3333333333333333703, 0.3170188387650512141, 0.3333333333333333703, 0.3170188387650512141, 0.3333333333333333703, 0.3170188387650512141, 0.3333333333333333703, 0.3170188387650512141, 0.3333333333333333703, 0.3170188387650512141, 0.3333333333333333703, 0.3170188387650512141, 0.3333333333333333703, 0.3170188387650512141, 0.3333333333333333703, 0.3170188387650512141, 0.3333333333333333703, 0.3170188387650512141, 0.3333333333333333703, 0.3170188387650512141, 0.3333333333333333703, 0.3170188387650512141, 0.3333333333333333703, 0.3170188387650512141, 0.3333333333333333703, 0.3170188387650512141, 0.3333333333333333703, 0.3170188387650512141, 0.3333333333333333703, 0.3170188387650512141, 0.3333333333333333703, 0.3170188387650512141, 0.3333333333333333703, 0.3170188387650512141, 0.3333333333333333703, 0.3170188387650512141, 0.3333333333333333703, 0.3170188387650512141, 0.3333333333333333703, 0.3170188387650512141, 0.3333333333333333703, 0.3170188387650512141, 0.3333333333333333703, 0.3170188387650512141, 0.3333333333333333703, 0.3170188387650512141, 0.3333333333333333703, 0.3170188387650512141, 0.3333333333333333703, 0.3170188387650512141, 0.3333333333333333703, 0.3170188387650512141, 0.3333333333333333703, 0.3170188387650512141, 0.3333333333333333703, 0.3170188387650512141, 0.3333333333333333703, 0.3170188387650512141, 0.3333333333333333703, 0.3170188387650512141, 0.3333333333333333703, 0.3170188387650512141, 0.3333333333333333703, 0.3170188387650512141, 0.3333333333333333703, 0.3170188387650512141, 0.3333333333333333703, 0.3170188387650512141, 0.3333333333333333703, 0.3170188387650512141, 0.3333333333333333703, 0.3170188387650512141, 0.3333333333333333703, 0.3170188387650512141, 0.3333333333333333703, 0.3170188387650512141, 0.3333333333333333703, 0.3170188387650512141, 0.3333333333333333703, 0.3170188387650512141, 0.3333333333333333703, 0.3170188387650512141, 0.3333333333333333703, 0.3170188387650512141, 0.3333333333333333703, 0.3170188387650512141, 0.3333333333333333703, 0.3170188387650512141, 0.3333333333333333703, 0.3170188387650512141, 0.3333333333333333703, 0.3170188387650512141, 0.3333333333333333703, 0.3170188387650512141, 0.3333333333333333703, 0.3170188387650512141, 0.3333333333333333703, 0.3170188387650512141, 0.3333333333333333703, 0.3170188387650512141, 0.3333333333333333703, 0.3170188387650512141, 0.3333333333333333703, 0.3170188387650512141, 0.3333333333333333703, 0.3170188387650512141, 0.3333333333333333703, 0.3170188387650512141, 0.3333333333333333703, 0.3170188387650512141, 0.3333333333333333703, 0.3170188387650512141, 0.3333333333333333703, 0.3170188387650512141, 0.3333333333333333703, 0.3170188387650512141, 0.3333333333333333703, 0.3170188387650512141, 0.3333333333333333703, 0.3170188387650512141, 0.3333333333333333703, 0.3170188387650512141, 0.3333333333333333703, 0.3170188387650512141, 0.3333333333333333703, 0.3170188387650512141, 0.3333333333333333703, 0.3170188387650512141, 0.3333333333333333703, 0.3170188387650512141, 0.3333333333333333703, 0.3170188387650512141, 0.3333333333333333703, 0.3170188387650512141, 0.3333333333333333703, 0.3170188387650512141, 0.3333333333333333703, 0.3170188387650512141, 0.3333333333333333703, 0.3170188387650512141, 0.3333333333333333703),
 ( 1.000000000000000000, 0.9510565162951535312, 1.000000000000000000, 0.9510565162951535312, 1.000000000000000000, 0.9510565162951535312, 1.000000000000000000, 0.9510565162951535312, 1.000000000000000000, 0.9510565162951535312, 1.000000000000000000, 0.9510565162951535312, 1.000000000000000000, 0.9510565162951535312, 1.000000000000000000, 0.9510565162951535312, 1.000000000000000000, 0.9510565162951535312, 1.000000000000000000, 0.9510565162951535312, 1.000000000000000000, 0.9510565162951535312, 1.000000000000000000, 0.9510565162951535312, 1.000000000000000000, 0.9510565162951535312, 1.000000000000000000, 0.9510565162951535312, 1.000000000000000000, 0.9510565162951535312, 1.000000000000000000, 0.9510565162951535312, 1.000000000000000000, 0.9510565162951535312, 1.000000000000000000, 0.9510565162951535312, 1.000000000000000000, 0.9510565162951535312, 1.000000000000000000, 0.9510565162951535312, 1.000000000000000000, 0.9510565162951535312, 1.000000000000000000, 0.9510565162951535312, 1.000000000000000000, 0.9510565162951535312, 1.000000000000000000, 0.9510565162951535312, 1.000000000000000000, 0.9510565162951535312, 1.000000000000000000, 0.9510565162951535312, 1.000000000000000000, 0.9510565162951535312, 1.000000000000000000, 0.9510565162951535312, 1.000000000000000000, 0.9510565162951535312, 1.000000000000000000, 0.9510565162951535312, 1.000000000000000000, 0.9510565162951535312, 1.000000000000000000, 0.9510565162951535312, 1.000000000000000000, 0.9510565162951535312, 1.000000000000000000, 0.9510565162951535312, 1.000000000000000000, 0.9510565162951535312, 1.000000000000000000, 0.9510565162951535312, 1.000000000000000000, 0.9510565162951535312, 1.000000000000000000, 0.9510565162951535312, 1.000000000000000000, 0.9510565162951535312, 1.000000000000000000, 0.9510565162951535312, 1.000000000000000000, 0.9510565162951535312, 1.000000000000000000, 0.9510565162951535312, 1.000000000000000000, 0.9510565162951535312, 1.000000000000000000, 0.9510565162951535312, 1.000000000000000000, 0.9510565162951535312, 1.000000000000000000, 0.9510565162951535312, 1.000000000000000000, 0.9510565162951535312, 1.000000000000000000, 0.9510565162951535312, 1.000000000000000000, 0.9510565162951535312, 1.000000000000000000, 0.9510565162951535312, 1.000000000000000000, 0.9510565162951535312, 1.000000000000000000, 0.9510565162951535312, 1.000000000000000000, 0.9510565162951535312, 1.000000000000000000, 0.9510565162951535312, 1.000000000000000000, 0.9510565162951535312, 1.000000000000000000, 0.9510565162951535312, 1.000000000000000000, 0.9510565162951535312, 1.000000000000000000, 0.9510565162951535312, 1.000000000000000000, 0.9510565162951535312, 1.000000000000000000, 0.9510565162951535312, 1.000000000000000000, 0.9510565162951535312, 1.000000000000000000, 0.9510565162951535312, 1.000000000000000000, 0.9510565162951535312, 1.000000000000000000, 0.9510565162951535312, 1.000000000000000000, 0.9510565162951535312, 1.000000000000000000, 0.9510565162951535312, 1.000000000000000000, 0.9510565162951535312, 1.000000000000000000, 0.9510565162951535312, 1.000000000000000000, 0.9510565162951535312, 1.000000000000000000, 0.9510565162951535312, 1.000000000000000000),
 ( 0.3333333333333333703, 0.3170188387650512141, 0.3333333333333333703, 0.3170188387650512141, 0.3333333333333333703, 0.3170188387650512141, 0.3333333333333333703, 0.3170188387650512141, 0.3333333333333333703, 0.3170188387650512141, 0.3333333333333333703, 0.3170188387650512141, 0.3333333333333333703, 0.3170188387650512141, 0.3333333333333333703, 0.3170188387650512141, 0.3333333333333333703, 0.3170188387650512141, 0.3333333333333333703, 0.3170188387650512141, 0.3333333333333333703, 0.3170188387650512141, 0.3333333333333333703, 0.3170188387650512141, 0.3333333333333333703, 0.3170188387650512141, 0.3333333333333333703, 0.3170188387650512141, 0.3333333333333333703, 0.3170188387650512141, 0.3333333333333333703, 0.3170188387650512141, 0.3333333333333333703, 0.3170188387650512141, 0.3333333333333333703, 0.3170188387650512141, 0.3333333333333333703, 0.3170188387650512141, 0.3333333333333333703, 0.3170188387650512141, 0.3333333333333333703, 0.3170188387650512141, 0.3333333333333333703, 0.3170188387650512141, 0.3333333333333333703, 0.3170188387650512141, 0.3333333333333333703, 0.3170188387650512141, 0.3333333333333333703, 0.3170188387650512141, 0.3333333333333333703, 0.3170188387650512141, 0.3333333333333333703, 0.3170188387650512141, 0.3333333333333333703, 0.3170188387650512141, 0.3333333333333333703, 0.3170188387650512141, 0.3333333333333333703, 0.3170188387650512141, 0.3333333333333333703, 0.3170188387650512141, 0.3333333333333333703, 0.3170188387650512141, 0.3333333333333333703, 0.3170188387650512141, 0.3333333333333333703, 0.3170188387650512141, 0.3333333333333333703, 0.3170188387650512141, 0.3333333333333333703, 0.3170188387650512141, 0.3333333333333333703, 0.3170188387650512141, 0.3333333333333333703, 0.3170188387650512141, 0.3333333333333333703, 0.3170188387650512141, 0.3333333333333333703, 0.3170188387650512141, 0.3333333333333333703, 0.3170188387650512141, 0.3333333333333333703, 0.3170188387650512141, 0.3333333333333333703, 0.3170188387650512141, 0.3333333333333333703, 0.3170188387650512141, 0.3333333333333333703, 0.3170188387650512141, 0.3333333333333333703, 0.3170188387650512141, 0.3333333333333333703, 0.3170188387650512141, 0.3333333333333333703, 0.3170188387650512141, 0.3333333333333333703, 0.3170188387650512141, 0.3333333333333333703, 0.3170188387650512141, 0.3333333333333333703, 0.3170188387650512141, 0.3333333333333333703, 0.3170188387650512141, 0.3333333333333333703, 0.3170188387650512141, 0.3333333333333333703, 0.3170188387650512141, 0.3333333333333333703, 0.3170188387650512141, 0.3333333333333333703, 0.3170188387650512141, 0.3333333333333333703, 0.3170188387650512141, 0.3333333333333333703, 0.3170188387650512141, 0.3333333333333333703, 0.3170188387650512141, 0.3333333333333333703, 0.3170188387650512141, 0.3333333333333333703, 0.3170188387650512141, 0.3333333333333333703, 0.3170188387650512141, 0.3333333333333333703, 0.3170188387650512141, 0.3333333333333333703, 0.3170188387650512141, 0.3333333333333333703, 0.3170188387650512141, 0.3333333333333333703, 0.3170188387650512141, 0.3333333333333333703, 0.3170188387650512141, 0.3333333333333333703, 0.3170188387650512141, 0.3333333333333333703, 0.3170188387650512141, 0.3333333333333333703, 0.3170188387650512141, 0.3333333333333333703),
 ( 0.3333333333333333703, 0.3170188387650512141, 0.3333333333333333703, 0.3170188387650512141, 0.3333333333333333703, 0.3170188387650512141, 0.3333333333333333703, 0.3170188387650512141, 0.3333333333333333703, 0.3170188387650512141, 0.3333333333333333703, 0.3170188387650512141, 0.3333333333333333703, 0.3170188387650512141, 0.3333333333333333703, 0.3170188387650512141, 0.3333333333333333703, 0.3170188387650512141, 0.3333333333333333703, 0.3170188387650512141, 0.3333333333333333703, 0.3170188387650512141, 0.3333333333333333703, 0.3170188387650512141, 0.3333333333333333703, 0.3170188387650512141, 0.3333333333333333703, 0.3170188387650512141, 0.3333333333333333703, 0.3170188387650512141, 0.3333333333333333703, 0.3170188387650512141, 0.3333333333333333703, 0.3170188387650512141, 0.3333333333333333703, 0.3170188387650512141, 0.3333333333333333703, 0.3170188387650512141, 0.3333333333333333703, 0.3170188387650512141, 0.3333333333333333703, 0.3170188387650512141, 0.3333333333333333703, 0.3170188387650512141, 0.3333333333333333703, 0.3170188387650512141, 0.3333333333333333703, 0.3170188387650512141, 0.3333333333333333703, 0.3170188387650512141, 0.3333333333333333703, 0.3170188387650512141, 0.3333333333333333703, 0.3170188387650512141, 0.3333333333333333703, 0.3170188387650512141, 0.3333333333333333703, 0.3170188387650512141, 0.3333333333333333703, 0.3170188387650512141, 0.3333333333333333703, 0.3170188387650512141, 0.3333333333333333703, 0.3170188387650512141, 0.3333333333333333703, 0.3170188387650512141, 0.3333333333333333703, 0.3170188387650512141, 0.3333333333333333703, 0.3170188387650512141, 0.3333333333333333703, 0.3170188387650512141, 0.3333333333333333703, 0.3170188387650512141, 0.3333333333333333703, 0.3170188387650512141, 0.3333333333333333703, 0.3170188387650512141, 0.3333333333333333703, 0.3170188387650512141, 0.3333333333333333703, 0.3170188387650512141, 0.3333333333333333703, 0.3170188387650512141, 0.3333333333333333703, 0.3170188387650512141, 0.3333333333333333703, 0.3170188387650512141, 0.3333333333333333703, 0.3170188387650512141, 0.3333333333333333703, 0.3170188387650512141, 0.3333333333333333703, 0.3170188387650512141, 0.3333333333333333703, 0.3170188387650512141, 0.3333333333333333703, 0.3170188387650512141, 0.3333333333333333703, 0.3170188387650512141, 0.3333333333333333703, 0.3170188387650512141, 0.3333333333333333703, 0.3170188387650512141, 0.3333333333333333703, 0.3170188387650512141, 0.3333333333333333703, 0.3170188387650512141, 0.3333333333333333703, 0.3170188387650512141, 0.3333333333333333703, 0.3170188387650512141, 0.3333333333333333703, 0.3170188387650512141, 0.3333333333333333703, 0.3170188387650512141, 0.3333333333333333703, 0.3170188387650512141, 0.3333333333333333703, 0.3170188387650512141, 0.3333333333333333703, 0.3170188387650512141, 0.3333333333333333703, 0.3170188387650512141, 0.3333333333333333703, 0.3170188387650512141, 0.3333333333333333703, 0.3170188387650512141, 0.3333333333333333703, 0.3170188387650512141, 0.3333333333333333703, 0.3170188387650512141, 0.3333333333333333703, 0.3170188387650512141, 0.3333333333333333703, 0.3170188387650512141, 0.3333333333333333703, 0.3170188387650512141, 0.3333333333333333703, 0.3170188387650512141, 0.3333333333333333703),
 ( 1.000000000000000000, 0.9510565162951535312, 1.000000000000000000, 0.9510565162951535312, 1.000000000000000000, 0.9510565162951535312, 1.000000000000000000, 0.9510565162951535312, 1.000000000000000000, 0.9510565162951535312, 1.000000000000000000, 0.9510565162951535312, 1.000000000000000000, 0.9510565162951535312, 1.000000000000000000, 0.9510565162951535312, 1.000000000000000000, 0.9510565162951535312, 1.000000000000000000, 0.9510565162951535312, 1.000000000000000000, 0.9510565162951535312, 1.000000000000000000, 0.9510565162951535312, 1.000000000000000000, 0.9510565162951535312, 1.000000000000000000, 0.9510565162951535312, 1.000000000000000000, 0.9510565162951535312, 1.000000000000000000, 0.9510565162951535312, 1.000000000000000000, 0.9510565162951535312, 1.000000000000000000, 0.9510565162951535312, 1.000000000000000000, 0.9510565162951535312, 1.000000000000000000, 0.9510565162951535312, 1.000000000000000000, 0.9510565162951535312, 1.000000000000000000, 0.9510565162951535312, 1.000000000000000000, 0.9510565162951535312, 1.000000000000000000, 0.9510565162951535312, 1.000000000000000000, 0.9510565162951535312, 1.000000000000000000, 0.9510565162951535312, 1.000000000000000000, 0.9510565162951535312, 1.000000000000000000, 0.9510565162951535312, 1.000000000000000000, 0.9510565162951535312, 1.000000000000000000, 0.9510565162951535312, 1.000000000000000000, 0.9510565162951535312, 1.000000000000000000, 0.9510565162951535312, 1.000000000000000000, 0.9510565162951535312, 1.000000000000000000, 0.9510565162951535312, 1.000000000000000000, 0.9510565162951535312, 1.000000000000000000, 0.9510565162951535312, 1.000000000000000000, 0.9510565162951535312, 1.000000000000000000, 0.9510565162951535312, 1.000000000000000000, 0.9510565162951535312, 1.000000000000000000, 0.9510565162951535312, 1.000000000000000000, 0.9510565162951535312, 1.000000000000000000, 0.9510565162951535312, 1.000000000000000000, 0.9510565162951535312, 1.000000000000000000, 0.9510565162951535312, 1.000000000000000000, 0.9510565162951535312, 1.000000000000000000, 0.9510565162951535312, 1.000000000000000000, 0.9510565162951535312, 1.000000000000000000, 0.9510565162951535312, 1.000000000000000000, 0.9510565162951535312, 1.000000000000000000, 0.9510565162951535312, 1.000000000000000000, 0.9510565162951535312, 1.000000000000000000, 0.9510565162951535312, 1.000000000000000000, 0.9510565162951535312, 1.000000000000000000, 0.9510565162951535312, 1.000000000000000000, 0.9510565162951535312, 1.000000000000000000, 0.9510565162951535312, 1.000000000000000000, 0.9510565162951535312, 1.000000000000000000, 0.9510565162951535312, 1.000000000000000000, 0.9510565162951535312, 1.000000000000000000, 0.9510565162951535312, 1.000000000000000000, 0.9510565162951535312, 1.000000000000000000, 0.9510565162951535312, 1.000000000000000000, 0.9510565162951535312, 1.000000000000000000, 0.9510565162951535312, 1.000000000000000000, 0.9510565162951535312, 1.000000000000000000, 0.9510565162951535312, 1.000000000000000000, 0.9510565162951535312, 1.000000000000000000, 0.9510565162951535312, 1.000000000000000000, 0.9510565162951535312, 1.000000000000000000, 0.9510565162951535312, 1.000000000000000000) ) ) 
 REPRESENTATION_ITEM ( '' )  SURFACE ( )  );
#6203=CARTESIAN_POINT ( 'NONE',  ( -34.10713997105786888, -31.14859572486944828, -7.938018618334151455 ) ) ;
#6204=CARTESIAN_POINT ( 'NONE',  ( -28.43739315969223824, -30.44999999999999574, -9.865911304835512041 ) ) ;
#6206=CARTESIAN_POINT ( 'NONE',  ( -25.46513832392765408, -46.65000000000001279, 8.900167166472096270 ) ) ;
#6213=CARTESIAN_POINT ( 'NONE',  ( -21.16389173201424612, -39.05140427513057944, -1.343104241417630185 ) ) ;
#6218=CARTESIAN_POINT ( 'NONE',  ( -28.60187809025093841, -45.45000000000000284, -8.827394325379140483 ) ) ;
#6224=CARTESIAN_POINT ( 'NONE',  ( -37.57355545560112375, -38.40000000000000568, 3.858919247786223305 ) ) ;
#6228=CARTESIAN_POINT ( 'NONE',  ( -31.50758917197619979, -44.94859572486942767, 9.874625247442176956 ) ) ;
#6231=CARTESIAN_POINT ( 'NONE',  ( -20.61696076434619584, -31.20000000000000639, 1.486127417882100676 ) ) ;
#6237=CARTESIAN_POINT ( 'NONE',  ( -36.04786814110010340, -42.99859572486943904, -5.972947139071243861 ) ) ;
#6238=CARTESIAN_POINT ( 'NONE',  ( -21.09983283352784156, -31.34999999999999787, 4.534861676072186043 ) ) ;
#6239=CARTESIAN_POINT ( 'NONE',  ( -21.12512167993187973, -48.35140427513057659, 4.584493831696868860 ) ) ;
#6248=DIRECTION ( 'NONE',  ( 0.7061138087190598212, -0.05297714858780431385, -0.7061138087190823587 ) ) ;
#6252=CARTESIAN_POINT ( 'NONE',  ( -34.10713997105786888, -46.14859572486944472, -7.938018618334151455 ) ) ;
#6253=CARTESIAN_POINT ( 'NONE',  ( -23.28248557872775137, -43.50000000000001421, 6.717514421272141156 ) ) ;
#6255=ADVANCED_FACE ( 'NONE', ( #1106 ), #5569, .T. ) ;
#6256=CARTESIAN_POINT ( 'NONE',  ( -23.28248557872775137, -46.50000000000000711, 6.717514421272141156 ) ) ;
#6260=CARTESIAN_POINT ( 'NONE',  ( -23.28248557872775137, -49.50000000000000711, 6.717514421272141156 ) ) ;
#6263=CARTESIAN_POINT ( 'NONE',  ( -38.38706344316003793, -46.70140427513057801, -1.382017864820032083 ) ) ;
#6265=CARTESIAN_POINT ( 'NONE',  ( -33.85891924778610473, -50.10000000000000853, 7.573555455601171715 ) ) ;
#6268=CARTESIAN_POINT ( 'NONE',  ( -36.31971658582311591, -35.24999999999998579, 6.319716585823199395 ) ) ;
#6271=CARTESIAN_POINT ( 'NONE',  ( -25.68709025247441602, -33.60000000000000142, -8.464561979789547053 ) ) ;
#6273=CARTESIAN_POINT ( 'NONE',  ( -22.93678734525658314, -42.75000000000000711, -7.063212654743582064 ) ) ;
#6277=CARTESIAN_POINT ( 'NONE',  ( -38.81868038277247734, -39.54859572486944330, 1.453139578080855365 ) ) ;
#6279=CARTESIAN_POINT ( 'NONE',  ( -20.13408869516453947, -31.05000000000000782, -1.562606840307983136 ) ) ;
#6280=CARTESIAN_POINT ( 'NONE',  ( -31.61762450863942320, -48.95140427513057091, 9.857197362228843573 ) ) ;
#6289=CARTESIAN_POINT ( 'NONE',  ( -31.38201786482021305, -43.29859572486943620, -8.387063443159975762 ) ) ;
#6290=CARTESIAN_POINT ( 'NONE',  ( -22.93678734525658314, -39.74999999999999289, -7.063212654743582952 ) ) ;
#6292=CARTESIAN_POINT ( 'NONE',  ( -38.90016716647221529, -50.84999999999999432, -4.534861676072185155 ) ) ;
#6297=CARTESIAN_POINT ( 'NONE',  ( -31.56260684030781505, -49.95000000000000995, 9.865911304835510265 ) ) ;
#6302=CARTESIAN_POINT ( 'NONE',  ( -34.05750781543318340, -33.15000000000001279, -7.963307464738195840 ) ) ;
#6308=FILL_AREA_STYLE ('',( #3587 ) ) ;
#6309=CARTESIAN_POINT ( 'NONE',  ( -22.03669253526174998, -37.35000000000000853, 4.057507815433014642 ) ) ;
#6313=CARTESIAN_POINT ( 'NONE',  ( -25.68709025247441602, -36.60000000000000853, -8.464561979789547053 ) ) ;
#6315=CARTESIAN_POINT ( 'NONE',  ( -23.28248557872775137, -40.50000000000000711, 6.717514421272141156 ) ) ;
#6316=( NAMED_UNIT ( * ) PLANE_ANGLE_UNIT ( ) SI_UNIT ( $, .RADIAN. ) );
#6320=CARTESIAN_POINT ( 'NONE',  ( -28.61798213517984024, -38.79859572486943620, 8.387063443159973986 ) ) ;
#6321=CARTESIAN_POINT ( 'NONE',  ( -20.14280263777121149, -50.04859572486944330, -1.617624508639600833 ) ) ;
#6322=CARTESIAN_POINT ( 'NONE',  ( -20.12537475255788522, -48.05140427513057233, -1.507589171976365439 ) ) ;
#6330=CARTESIAN_POINT ( 'NONE',  ( -21.18131961722757595, -44.04859572486944330, -1.453139578080854699 ) ) ;
#6331=CARTESIAN_POINT ( 'NONE',  ( -21.09983283352784156, -40.35000000000000142, 4.534861676072186043 ) ) ;
#6334=CARTESIAN_POINT ( 'NONE',  ( -34.31290974752564438, -44.10000000000000853, 8.464561979789547053 ) ) ;
#6344=CARTESIAN_POINT ( 'NONE',  ( -31.39812190974910422, -34.95000000000000995, 8.827394325379140483 ) ) ;
#6352=CARTESIAN_POINT ( 'NONE',  ( -23.98959235991431171, -34.50000000000000000, 6.010407640085604797 ) ) ;
#6355=CARTESIAN_POINT ( 'NONE',  ( -23.28248557872775137, -37.50000000000000711, 6.717514421272141156 ) ) ;
#6357=CARTESIAN_POINT ( 'NONE',  ( -31.56260684030781505, -43.95000000000000284, 9.865911304835508489 ) ) ;
#6361=CARTESIAN_POINT ( 'NONE',  ( -26.18828373723858149, -37.59859572486943335, -7.597606577763319713 ) ) ;
#6362=CARTESIAN_POINT ( 'NONE',  ( -21.07454398712378918, -47.34859572486942625, 4.485229520447505003 ) ) ;
#6364=CARTESIAN_POINT ( 'NONE',  ( -28.56619749409589204, -48.80140427513057233, 9.391326687552490782 ) ) ;
#6367=CARTESIAN_POINT ( 'NONE',  ( -25.68709025247441602, -33.60000000000000142, -8.464561979789547053 ) ) ;
#6374=CARTESIAN_POINT ( 'NONE',  ( -22.45049566656107842, -43.89859572486944472, -3.906122232810846917 ) ) ;
#6375=CARTESIAN_POINT ( 'NONE',  ( -21.09983283352784156, -43.35000000000000853, 4.534861676072186043 ) ) ;
#6378=CARTESIAN_POINT ( 'NONE',  ( -23.31994607974211675, -39.50140427513058228, 6.754974922286503869 ) ) ;
#6386=CARTESIAN_POINT ( 'NONE',  ( -37.96330746473829976, -35.84999999999998721, -4.057507815433013754 ) ) ;
#6396=CARTESIAN_POINT ( 'NONE',  ( -31.39812190974910422, -43.95000000000000284, 8.827394325379140483 ) ) ;
#6401=CARTESIAN_POINT ( 'NONE',  ( -39.38303923565386100, -38.70000000000000284, -1.486127417882099788 ) ) ;
#6403=CARTESIAN_POINT ( 'NONE',  ( -38.90016716647221529, -41.85000000000000142, -4.534861676072185155 ) ) ;
#6406=CARTESIAN_POINT ( 'NONE',  ( -37.98859631114233792, -51.84859572486944757, -4.007875659808334490 ) ) ;
#6407=CARTESIAN_POINT ( 'NONE',  ( -22.93678734525658314, -30.75000000000000000, -7.063212654743582952 ) ) ;
#6408=CARTESIAN_POINT ( 'NONE',  ( -38.87487832006816291, -49.85140427513058370, -4.584493831696867971 ) ) ;
#6411=CARTESIAN_POINT ( 'NONE',  ( -20.13408869516453947, -40.05000000000001137, -1.562606840307983136 ) ) ;
#6412=DIRECTION ( 'NONE',  ( 0.7071067811865556774, 0.000000000000000000, 0.7071067811865392461 ) ) ;
#6417=CARTESIAN_POINT ( 'NONE',  ( -37.54950433343896776, -39.39859572486943762, 3.906122232810848249 ) ) ;
#6418=CARTESIAN_POINT ( 'NONE',  ( -28.43739315969223824, -48.44999999999999574, -9.865911304835512041 ) ) ;
#6421=CARTESIAN_POINT ( 'NONE',  ( -22.89739904353894318, -32.75140427513057517, -7.023824353025938549 ) ) ;
#6431=CARTESIAN_POINT ( 'NONE',  ( -25.94249218456686279, -37.65000000000000568, 7.963307464738195840 ) ) ;
#6434=UNCERTAINTY_MEASURE_WITH_UNIT (LENGTH_MEASURE( 1.000000000000000082E-05 ), #6932, 'distance_accuracy_value', 'NONE');
#6445=CARTESIAN_POINT ( 'NONE',  ( -20.13408869516454303, -37.05000000000000426, -1.562606840307982692 ) ) ;
#6447=CARTESIAN_POINT ( 'NONE',  ( -36.04786814110010340, -45.99859572486943904, -5.972947139071243861 ) ) ;
#6448=CARTESIAN_POINT ( 'NONE',  ( -28.43739315969223824, -36.45000000000000284, -9.865911304835512041 ) ) ;
#6449=CARTESIAN_POINT ( 'NONE',  ( -26.09387776718931917, -38.60140427513057659, -7.549504333439021941 ) ) ;
#6452=CARTESIAN_POINT ( 'NONE',  ( -25.68709025247441602, -36.60000000000000853, -8.464561979789547053 ) ) ;
#6459=CARTESIAN_POINT ( 'NONE',  ( -34.10713997105786888, -49.14859572486945183, -7.938018618334151455 ) ) ;
#6460=CARTESIAN_POINT ( 'NONE',  ( -22.89739904353894318, -32.75140427513057517, -7.023824353025938549 ) ) ;
#6462=CARTESIAN_POINT ( 'NONE',  ( -20.12537475255788522, -39.05140427513057944, -1.507589171976365439 ) ) ;
#6469=CARTESIAN_POINT ( 'NONE',  ( -36.01040764008574513, -36.00000000000000711, -6.010407640085605685 ) ) ;
#6485=PRESENTATION_STYLE_ASSIGNMENT (( #3027 ) ) ;
#6487=CARTESIAN_POINT ( 'NONE',  ( -21.55948914237271907, -31.89859572486943762, -4.360112732550413206 ) ) ;
#6488=CARTESIAN_POINT ( 'NONE',  ( -22.93678734525658314, -36.75000000000000711, -7.063212654743582952 ) ) ;
#6489=CARTESIAN_POINT ( 'NONE',  ( -34.00787565980851213, -35.15140427513058086, -7.988596311142238449 ) ) ;
#6493=CARTESIAN_POINT ( 'NONE',  ( -25.73429323749904185, -37.59859572486943335, -8.488613101951701267 ) ) ;
#6494=CARTESIAN_POINT ( 'NONE',  ( -39.86591130483550671, -32.55000000000000426, 1.562606840307984468 ) ) ;
#6499=CARTESIAN_POINT ( 'NONE',  ( -33.81171626276147890, -48.09859572486944046, 7.597606577763319713 ) ) ;
#6500=CARTESIAN_POINT ( 'NONE',  ( -28.56619749409589204, -30.80140427513057233, 9.391326687552490782 ) ) ;
#6504=CARTESIAN_POINT ( 'NONE',  ( -37.10260095646111012, -34.25140427513057517, 7.023824353025939438 ) ) ;
#6512=CARTESIAN_POINT ( 'NONE',  ( -23.98959235991431171, -43.50000000000001421, 6.010407640085604797 ) ) ;
#6518=CARTESIAN_POINT ( 'NONE',  ( -22.06198138166579170, -33.35140427513057659, 4.107139971057695682 ) ) ;
#6524=CARTESIAN_POINT ( 'NONE',  ( -33.85891924778610473, -35.10000000000000853, 7.573555455601171715 ) ) ;
#6527=CARTESIAN_POINT ( 'NONE',  ( -23.28248557872775137, -46.50000000000000711, 6.717514421272141156 ) ) ;
#6530=CARTESIAN_POINT ( 'NONE',  ( -31.38201786482021305, -46.29859572486944330, -8.387063443159975762 ) ) ;
#6531=CARTESIAN_POINT ( 'NONE',  ( -34.31290974752564438, -35.10000000000000853, 8.464561979789547053 ) ) ;
#6532=CARTESIAN_POINT ( 'NONE',  ( -31.45313957808072303, -39.95140427513058512, 8.818680382772479120 ) ) ;
#6535=CARTESIAN_POINT ( 'NONE',  ( -28.46154767013959486, -35.79859572486943620, 9.374751783755112200 ) ) ;
#6536=CARTESIAN_POINT ( 'NONE',  ( -23.28248557872775137, -34.50000000000000000, 6.717514421272141156 ) ) ;
#6542=CARTESIAN_POINT ( 'NONE',  ( -20.14280263777121149, -32.04859572486944330, -1.617624508639600833 ) ) ;
#6543=CARTESIAN_POINT ( 'NONE',  ( -37.10260095646111012, -31.25140427513058228, 7.023824353025939438 ) ) ;
#6546=CARTESIAN_POINT ( 'NONE',  ( -31.43380250590416125, -38.30140427513057944, -9.391326687552492558 ) ) ;
#6554=CARTESIAN_POINT ( 'NONE',  ( -28.67030704715798350, -37.80000000000000426, 8.395350895058669494 ) ) ;
#6560=CARTESIAN_POINT ( 'NONE',  ( -31.48612741788231517, -39.30000000000001137, -9.383039235653804155 ) ) ;
#6563=CARTESIAN_POINT ( 'NONE',  ( -33.90612223281073057, -37.10140427513057659, 7.549504333439023718 ) ) ;
#6566=CARTESIAN_POINT ( 'NONE',  ( -26.14108075221394856, -36.60000000000000853, -7.573555455601170827 ) ) ;
#6571=CARTESIAN_POINT ( 'NONE',  ( -37.98859631114233792, -45.84859572486944046, -4.007875659808334490 ) ) ;
#6572=CARTESIAN_POINT ( 'NONE',  ( -28.51387258211773812, -37.80000000000000426, 9.383039235653802379 ) ) ;
#6573=CARTESIAN_POINT ( 'NONE',  ( -38.38706344316003793, -34.70140427513057091, -1.382017864820032083 ) ) ;
#6576=CARTESIAN_POINT ( 'NONE',  ( -37.02382435302582309, -36.24859572486943904, 7.102600956461226467 ) ) ;
#6577=CARTESIAN_POINT ( 'NONE',  ( -20.13408869516453947, -43.04999999999999005, -1.562606840307983136 ) ) ;
#6584=CARTESIAN_POINT ( 'NONE',  ( -22.45049566656107842, -46.89859572486944472, -3.906122232810846917 ) ) ;
#6585=CARTESIAN_POINT ( 'NONE',  ( -36.68005392025794009, -29.00140427513058583, -6.754974922286504757 ) ) ;
#6588=CARTESIAN_POINT ( 'NONE',  ( -31.43380250590416125, -44.30140427513057944, -9.391326687552492558 ) ) ;
#6595=CARTESIAN_POINT ( 'NONE',  ( -21.17260567462091458, -43.04999999999999005, -1.398121909749242331 ) ) ;
#6600=CARTESIAN_POINT ( 'NONE',  ( -38.90016716647221529, -41.84999999999999432, -4.534861676072185155 ) ) ;
#6603=CARTESIAN_POINT ( 'NONE',  ( -38.83610826798580717, -37.55140427513057944, 1.343104241417631073 ) ) ;
#6607=CARTESIAN_POINT ( 'NONE',  ( -28.67030704715798350, -37.80000000000000426, 8.395350895058669494 ) ) ;
#6614=CARTESIAN_POINT ( 'NONE',  ( -39.38303923565386100, -38.70000000000000284, -1.486127417882099788 ) ) ;
#6615=CARTESIAN_POINT ( 'NONE',  ( -28.72263195913613387, -36.80140427513057944, 8.403638346957361449 ) ) ;
#6618=CARTESIAN_POINT ( 'NONE',  ( -37.02382435302582309, -33.24859572486943193, 7.102600956461226467 ) ) ;
#6625=CARTESIAN_POINT ( 'NONE',  ( -22.01140368885771892, -50.34859572486944046, 4.007875659808335378 ) ) ;
#6626=CARTESIAN_POINT ( 'NONE',  ( -39.87462524744216807, -31.55140427513057588, 1.507589171976367215 ) ) ;
#6630=CARTESIAN_POINT ( 'NONE',  ( -36.68005392025794009, -50.00140427513058938, -6.754974922286504757 ) ) ;
#6638=CARTESIAN_POINT ( 'NONE',  ( -36.01040764008574513, -45.00000000000000711, -6.010407640085605685 ) ) ;
#6644=CARTESIAN_POINT ( 'NONE',  ( -21.53543802021056663, -39.90000000000000568, -4.312909747525783821 ) ) ;
#6649=CARTESIAN_POINT ( 'NONE',  ( -26.09387776718931917, -35.60140427513057659, -7.549504333439021941 ) ) ;
#6653=CARTESIAN_POINT ( 'NONE',  ( -37.57355545560112375, -38.40000000000000568, 3.858919247786223305 ) ) ;
#6655=CARTESIAN_POINT ( 'NONE',  ( -25.68709025247441602, -48.60000000000000142, -8.464561979789547053 ) ) ;
#6660=CARTESIAN_POINT ( 'NONE',  ( -36.71751442127229836, -45.00000000000000711, -6.717514421272142044 ) ) ;
#6661=CARTESIAN_POINT ( 'NONE',  ( -28.54686042191934092, -44.45140427513058512, -8.818680382772479120 ) ) ;
#6665=CARTESIAN_POINT ( 'NONE',  ( -39.85719736222883824, -36.54859572486943620, 1.617624508639602388 ) ) ;
#6673=CARTESIAN_POINT ( 'NONE',  ( -33.85891924778610473, -50.10000000000000853, 7.573555455601171715 ) ) ;
#6674=CARTESIAN_POINT ( 'NONE',  ( -38.44051085762733777, -39.39859572486943762, 4.360112732550414982 ) ) ;
#6675=CARTESIAN_POINT ( 'NONE',  ( -31.43380250590416125, -44.30140427513057944, -9.391326687552492558 ) ) ;
#6678=CARTESIAN_POINT ( 'NONE',  ( -34.36011273255026310, -46.10140427513058370, 8.440510857627391061 ) ) ;
#6685=CARTESIAN_POINT ( 'NONE',  ( -25.94249218456686279, -43.64999999999999147, 7.963307464738195840 ) ) ;
#6691=CARTESIAN_POINT ( 'NONE',  ( -21.53543802021056663, -48.90000000000000568, -4.312909747525783821 ) ) ;
#6694=CARTESIAN_POINT ( 'NONE',  ( -36.35910488754074521, -34.25140427513057517, 6.280328284105565650 ) ) ;
#6697=CARTESIAN_POINT ( 'NONE',  ( -21.60464910494133406, -31.20000000000000639, 1.329692952841886155 ) ) ;
#6703=CARTESIAN_POINT ( 'NONE',  ( -39.86591130483550671, -47.54999999999999716, 1.562606840307984468 ) ) ;
#6704=CARTESIAN_POINT ( 'NONE',  ( -28.72263195913613387, -45.80140427513057944, 8.403638346957361449 ) ) ;
#6709=CARTESIAN_POINT ( 'NONE',  ( -34.26570676250101855, -45.09859572486944046, 8.488613101951703044 ) ) ;
#6717=CARTESIAN_POINT ( 'NONE',  ( -21.60464910494133406, -49.20000000000000995, 1.329692952841886155 ) ) ;
#6718=CARTESIAN_POINT ( 'NONE',  ( -39.39132668755255651, -36.69859572486944188, -1.433802505903950308 ) ) ;
#6719=CARTESIAN_POINT ( 'NONE',  ( -31.43380250590416125, -38.30140427513057944, -9.391326687552492558 ) ) ;
#6723=CARTESIAN_POINT ( 'NONE',  ( -39.37475178375516549, -46.70140427513057801, -1.538452329860249712 ) ) ;
#6731=CARTESIAN_POINT ( 'NONE',  ( -34.05750781543318340, -48.15000000000001279, -7.963307464738195840 ) ) ;
#6732=CARTESIAN_POINT ( 'NONE',  ( -31.48612741788231517, -36.30000000000000426, -9.383039235653804155 ) ) ;
#6733=EDGE_LOOP ( 'NONE', ( #377, #3524, #5043, #7206 ) ) ;
#6736=CARTESIAN_POINT ( 'NONE',  ( -38.46456197978948666, -44.40000000000000568, 4.312909747525784709 ) ) ;
#6739=CARTESIAN_POINT ( 'NONE',  ( -22.06198138166579170, -39.35140427513057659, 4.107139971057695682 ) ) ;
#6741=CARTESIAN_POINT ( 'NONE',  ( -37.96330746473829976, -41.85000000000000142, -4.057507815433013754 ) ) ;
#6746=CARTESIAN_POINT ( 'NONE',  ( -21.53543802021056663, -48.90000000000000568, -4.312909747525783821 ) ) ;
#6747=CARTESIAN_POINT ( 'NONE',  ( -28.72263195913613387, -48.80140427513057233, 8.403638346957361449 ) ) ;
#6751=CARTESIAN_POINT ( 'NONE',  ( -37.02382435302582309, -51.24859572486943193, 7.102600956461226467 ) ) ;
#6753=CARTESIAN_POINT ( 'NONE',  ( -31.48612741788231517, -33.30000000000000426, -9.383039235653804155 ) ) ;
#6756=CARTESIAN_POINT ( 'NONE',  ( -21.17260567462091458, -49.04999999999999716, -1.398121909749242331 ) ) ;
#6757=CARTESIAN_POINT ( 'NONE',  ( -23.24502507771338600, -35.49859572486943193, 6.680053920257780220 ) ) ;
#6758=CARTESIAN_POINT ( 'NONE',  ( -21.12512167993187973, -45.35140427513057659, 4.584493831696868860 ) ) ;
#6763=CARTESIAN_POINT ( 'NONE',  ( -38.48861310195163554, -43.40140427513058796, 4.265706762501153548 ) ) ;
#6770=CARTESIAN_POINT ( 'NONE',  ( -37.96330746473829976, -47.85000000000000853, -4.057507815433013754 ) ) ;
#6771=CARTESIAN_POINT ( 'NONE',  ( -31.56260684030781505, -37.94999999999998153, 9.865911304835510265 ) ) ;
#6777=CARTESIAN_POINT ( 'NONE',  ( -39.86591130483550671, -47.54999999999999716, 1.562606840307984468 ) ) ;
#6781=CARTESIAN_POINT ( 'NONE',  ( -21.61293655684001536, -45.20140427513059223, 1.382017864820032971 ) ) ;
#6785=CARTESIAN_POINT ( 'NONE',  ( -23.98959235991431171, -46.50000000000000711, 6.010407640085604797 ) ) ;
#6792=CARTESIAN_POINT ( 'NONE',  ( -25.46513832392765408, -43.64999999999999147, 8.900167166472096270 ) ) ;
#6793=CARTESIAN_POINT ( 'NONE',  ( -36.35910488754074521, -49.25140427513058938, 6.280328284105565650 ) ) ;
#6796=PRODUCT_DEFINITION ( 'UNKNOWN', '', #6074, #1772 ) ;
#6799=CARTESIAN_POINT ( 'NONE',  ( -28.46154767013959486, -44.79859572486943620, 9.374751783755112200 ) ) ;
#6802=CARTESIAN_POINT ( 'NONE',  ( -21.09983283352783801, -31.34999999999999432, 4.534861676072186043 ) ) ;
#6806=CARTESIAN_POINT ( 'NONE',  ( -31.34310424141748896, -32.94859572486944188, 8.836108267985801845 ) ) ;
#6807=CARTESIAN_POINT ( 'NONE',  ( -21.55948914237271907, -40.89859572486943762, -4.360112732550413206 ) ) ;
#6808=CARTESIAN_POINT ( 'NONE',  ( -25.63988726744978663, -38.60140427513057659, -8.440510857627391061 ) ) ;
#6818=CARTESIAN_POINT ( 'NONE',  ( -38.40363834695740053, -33.69859572486942767, -1.277368040863739118 ) ) ;
#6819=CARTESIAN_POINT ( 'NONE',  ( -25.68709025247441602, -30.60000000000000142, -8.464561979789547053 ) ) ;
#6824=CARTESIAN_POINT ( 'NONE',  ( -37.06321265474346660, -50.24999999999998579, 7.063212654743582952 ) ) ;
#6827=CARTESIAN_POINT ( 'NONE',  ( -22.40239342223677355, -41.90140427513058086, -3.811716262761597473 ) ) ;
#6830=CARTESIAN_POINT ( 'NONE',  ( -23.68028341417693738, -45.75000000000000000, -6.319716585823200283 ) ) ;
#6835=CARTESIAN_POINT ( 'NONE',  ( -34.31290974752564438, -47.10000000000000142, 8.464561979789547053 ) ) ;
#6836=CARTESIAN_POINT ( 'NONE',  ( -28.67030704715798350, -31.80000000000000782, 8.395350895058669494 ) ) ;
#6840=CARTESIAN_POINT ( 'NONE',  ( -21.07454398712378918, -44.34859572486944046, 4.485229520447505003 ) ) ;
#6842=CARTESIAN_POINT ( 'NONE',  ( -37.06321265474346660, -35.25000000000000000, 7.063212654743582952 ) ) ;
#6848=CARTESIAN_POINT ( 'NONE',  ( -23.95213185889994989, -38.49859572486943904, 5.972947139071243861 ) ) ;
#6849=CARTESIAN_POINT ( 'NONE',  ( -20.14280263777121149, -44.04859572486944330, -1.617624508639600833 ) ) ;
#6850=CARTESIAN_POINT ( 'NONE',  ( -34.48522952044771017, -38.15140427513058086, -8.925456012876139766 ) ) ;
#6854=CARTESIAN_POINT ( 'NONE',  ( -31.48612741788231517, -30.30000000000000782, -9.383039235653804155 ) ) ;
#6861=CARTESIAN_POINT ( 'NONE',  ( -37.54950433343896776, -36.39859572486944472, 3.906122232810848249 ) ) ;
#6862=CARTESIAN_POINT ( 'NONE',  ( -36.71751442127229836, -33.00000000000000711, -6.717514421272142044 ) ) ;
#6864=CARTESIAN_POINT ( 'NONE',  ( -37.06321265474346660, -50.24999999999998579, 7.063212654743582952 ) ) ;
#6871=CARTESIAN_POINT ( 'NONE',  ( -26.09387776718931917, -41.60140427513058370, -7.549504333439021941 ) ) ;
#6875=CARTESIAN_POINT ( 'NONE',  ( -37.96330746473829976, -47.85000000000000142, -4.057507815433013754 ) ) ;
#6880=CARTESIAN_POINT ( 'NONE',  ( -33.85891924778610473, -41.10000000000000142, 7.573555455601171715 ) ) ;
#6884=CARTESIAN_POINT ( 'NONE',  ( -31.53845232986046554, -49.29859572486945041, -9.374751783755117529 ) ) ;
#6886=CARTESIAN_POINT ( 'NONE',  ( -31.56260684030781505, -31.95000000000000639, 9.865911304835508489 ) ) ;
#6890=CARTESIAN_POINT ( 'NONE',  ( -21.18131961722757595, -41.04859572486944330, -1.453139578080854699 ) ) ;
#6892=CARTESIAN_POINT ( 'NONE',  ( -37.02382435302582309, -45.24859572486943904, 7.102600956461226467 ) ) ;
#6893=CARTESIAN_POINT ( 'NONE',  ( -34.36011273255026310, -49.10140427513058370, 8.440510857627391061 ) ) ;
#6904=CARTESIAN_POINT ( 'NONE',  ( -38.82739432537914581, -47.54999999999999716, 1.398121909749243441 ) ) ;
#6905=CARTESIAN_POINT ( 'NONE',  ( -31.48612741788231517, -30.30000000000000782, -9.383039235653804155 ) ) ;
#6908=CARTESIAN_POINT ( 'NONE',  ( -37.06321265474346660, -47.25000000000000711, 7.063212654743582952 ) ) ;
#6912=CARTESIAN_POINT ( 'NONE',  ( -36.71751442127229836, -51.00000000000000711, -6.717514421272142044 ) ) ;
#6915=CARTESIAN_POINT ( 'NONE',  ( -37.59760657776328685, -46.40140427513058086, 3.811716262761598362 ) ) ;
#6918=CARTESIAN_POINT ( 'NONE',  ( -23.98959235991431171, -49.50000000000000711, 6.010407640085604797 ) ) ;
#6924=CARTESIAN_POINT ( 'NONE',  ( -28.67030704715798350, -34.80000000000000426, 8.395350895058669494 ) ) ;
#6928=CARTESIAN_POINT ( 'NONE',  ( -21.09983283352784156, -34.35000000000000853, 4.534861676072186043 ) ) ;
#6930=CARTESIAN_POINT ( 'NONE',  ( -22.93678734525658314, -30.75000000000000000, -7.063212654743582064 ) ) ;
#6932=( LENGTH_UNIT ( ) NAMED_UNIT ( * ) SI_UNIT ( .MILLI., .METRE. ) );
#6937=CARTESIAN_POINT ( 'NONE',  ( -31.38201786482021305, -40.29859572486944330, -8.387063443159975762 ) ) ;
#6938=CARTESIAN_POINT ( 'NONE',  ( -25.46513832392765408, -31.65000000000000568, 8.900167166472096270 ) ) ;
#6939=CARTESIAN_POINT ( 'NONE',  ( -33.90612223281073057, -34.10140427513057659, 7.549504333439023718 ) ) ;
#6948=CARTESIAN_POINT ( 'NONE',  ( -28.65689575858256077, -37.44859572486943478, -8.836108267985801845 ) ) ;
#6950=CARTESIAN_POINT ( 'NONE',  ( -21.53543802021056663, -42.90000000000000568, -4.312909747525783821 ) ) ;
#6953=CARTESIAN_POINT ( 'NONE',  ( -36.68005392025794009, -29.00140427513058583, -6.754974922286504757 ) ) ;
#6960=CARTESIAN_POINT ( 'NONE',  ( -28.60187809025093841, -30.44999999999999574, -8.827394325379140483 ) ) ;
#6967=CARTESIAN_POINT ( 'NONE',  ( -31.39812190974910422, -34.95000000000000995, 8.827394325379140483 ) ) ;
#6970=EDGE_CURVE ( 'NONE', #282, #4270, #3707, .T. ) ;
#6972=CARTESIAN_POINT ( 'NONE',  ( -38.90016716647221529, -35.84999999999998721, -4.534861676072185155 ) ) ;
#6974=CARTESIAN_POINT ( 'NONE',  ( -25.46513832392766119, -40.65000000000000568, 8.900167166472096270 ) ) ;
#6978=CARTESIAN_POINT ( 'NONE',  ( -38.81868038277247734, -36.54859572486943620, 1.453139578080855365 ) ) ;
#6980=CARTESIAN_POINT ( 'NONE',  ( -31.53845232986046554, -49.29859572486945041, -9.374751783755117529 ) ) ;
#6981=CARTESIAN_POINT ( 'NONE',  ( -24.02705286092866643, -30.50140427513058583, 6.047868141099968398 ) ) ;
#6992=CARTESIAN_POINT ( 'NONE',  ( -22.01140368885771892, -41.34859572486944757, 4.007875659808335378 ) ) ;
#6993=CARTESIAN_POINT ( 'NONE',  ( -21.09983283352784156, -46.34999999999998721, 4.534861676072186043 ) ) ;
#6995=CARTESIAN_POINT ( 'NONE',  ( -25.46513832392765408, -49.64999999999999147, 8.900167166472096270 ) ) ;
#7001=CARTESIAN_POINT ( 'NONE',  ( -20.61696076434619584, -49.20000000000000995, 1.486127417882100676 ) ) ;
#7005=CARTESIAN_POINT ( 'NONE',  ( -22.42644454439892598, -33.90000000000000568, -3.858919247786222861 ) ) ;
#7012=CARTESIAN_POINT ( 'NONE',  ( -38.82739432537914581, -35.55000000000001137, 1.398121909749243441 ) ) ;
#7015=CARTESIAN_POINT ( 'NONE',  ( -31.56260684030781505, -34.95000000000000995, 9.865911304835510265 ) ) ;
#7018=CARTESIAN_POINT ( 'NONE',  ( -20.61696076434619584, -37.20000000000000284, 1.486127417882100676 ) ) ;
#7023=CARTESIAN_POINT ( 'NONE',  ( -25.89286002894218086, -41.64859572486943762, 7.938018618334153231 ) ) ;
#7024=CARTESIAN_POINT ( 'NONE',  ( -39.39132668755255651, -51.69859572486944188, -1.433802505903950308 ) ) ;
#7025=CARTESIAN_POINT ( 'NONE',  ( -39.87462524744216807, -46.55140427513058654, 1.507589171976367215 ) ) ;
#7036=CARTESIAN_POINT ( 'NONE',  ( -34.10713997105786888, -43.14859572486943762, -7.938018618334151455 ) ) ;
#7037=CARTESIAN_POINT ( 'NONE',  ( -37.06321265474346660, -41.25000000000000711, 7.063212654743582952 ) ) ;
#7039=CARTESIAN_POINT ( 'NONE',  ( -37.06321265474346660, -44.25000000000000000, 7.063212654743582952 ) ) ;
#7050=CARTESIAN_POINT ( 'NONE',  ( -23.98959235991431171, -34.50000000000000000, 6.010407640085604797 ) ) ;
#7059=CARTESIAN_POINT ( 'NONE',  ( -36.01040764008574513, -36.00000000000000711, -6.010407640085605685 ) ) ;
#7063=CARTESIAN_POINT ( 'NONE',  ( -22.42644454439892598, -30.90000000000000924, -3.858919247786222861 ) ) ;
#7064=CARTESIAN_POINT ( 'NONE',  ( -28.51387258211773812, -37.80000000000000426, 9.383039235653802379 ) ) ;
#7066=CARTESIAN_POINT ( 'NONE',  ( -21.09983283352783801, -43.35000000000000853, 4.534861676072186043 ) ) ;
#7067=SURFACE_SIDE_STYLE ('',( #278 ) ) ;
#7072=CARTESIAN_POINT ( 'NONE',  ( -36.04786814110010340, -48.99859572486944614, -5.972947139071243861 ) ) ;
#7073=CARTESIAN_POINT ( 'NONE',  ( -39.85719736222883824, -51.54859572486944330, 1.617624508639602388 ) ) ;
#7075=CARTESIAN_POINT ( 'NONE',  ( -38.87487832006816291, -46.85140427513056949, -4.584493831696867971 ) ) ;
#7078=CARTESIAN_POINT ( 'NONE',  ( -34.53486167607238144, -33.15000000000001279, -8.900167166472096270 ) ) ;
#7086=CARTESIAN_POINT ( 'NONE',  ( -28.61798213517984024, -44.79859572486943620, 8.387063443159973986 ) ) ;
#7087=CARTESIAN_POINT ( 'NONE',  ( -34.53486167607238144, -48.15000000000001279, -8.900167166472096270 ) ) ;
#7089=CARTESIAN_POINT ( 'NONE',  ( -34.36011273255026310, -34.10140427513057659, 8.440510857627391061 ) ) ;
#7096=CARTESIAN_POINT ( 'NONE',  ( -21.60464910494133406, -37.20000000000000284, 1.329692952841886155 ) ) ;
#7107=CARTESIAN_POINT ( 'NONE',  ( -31.56260684030781505, -31.95000000000000639, 9.865911304835510265 ) ) ;
#7109=CARTESIAN_POINT ( 'NONE',  ( -21.53543802021056663, -42.90000000000000568, -4.312909747525783821 ) ) ;
#7111=CARTESIAN_POINT ( 'NONE',  ( -23.95213185889994989, -47.49859572486944614, 5.972947139071243861 ) ) ;
#7112=CARTESIAN_POINT ( 'NONE',  ( -22.93678734525658314, -39.74999999999999289, -7.063212654743582952 ) ) ;
#7113=CARTESIAN_POINT ( 'NONE',  ( -23.64089511245930098, -41.75140427513057517, -6.280328284105564762 ) ) ;
#7117=CARTESIAN_POINT ( 'NONE',  ( -39.38303923565386100, -35.70000000000000995, -1.486127417882099788 ) ) ;
#7124=CARTESIAN_POINT ( 'NONE',  ( -36.04786814110010340, -45.99859572486943904, -5.972947139071243861 ) ) ;
#7125=CARTESIAN_POINT ( 'NONE',  ( -25.51477047955235378, -33.65140427513057375, 8.925456012876139766 ) ) ;
#7127=CARTESIAN_POINT ( 'NONE',  ( -39.87462524744216807, -34.55140427513057233, 1.507589171976367215 ) ) ;
#7135=CARTESIAN_POINT ( 'NONE',  ( -34.05750781543318340, -30.15000000000000213, -7.963307464738195840 ) ) ;
#7149=CARTESIAN_POINT ( 'NONE',  ( -36.71751442127229836, -45.00000000000000711, -6.717514421272142044 ) ) ;
#7150=( LENGTH_UNIT ( ) NAMED_UNIT ( * ) SI_UNIT ( .MILLI., .METRE. ) );
#7152=CARTESIAN_POINT ( 'NONE',  ( -21.07454398712378918, -32.34859572486942625, 4.485229520447505003 ) ) ;
#7153=CARTESIAN_POINT ( 'NONE',  ( -38.46456197978948666, -41.40000000000000568, 4.312909747525784709 ) ) ;
#7154=CARTESIAN_POINT ( 'NONE',  ( -33.90612223281073057, -43.10140427513058370, 7.549504333439023718 ) ) ;
#7158=CARTESIAN_POINT ( 'NONE',  ( -39.39132668755255651, -33.69859572486942767, -1.433802505903950308 ) ) ;
#7159=CARTESIAN_POINT ( 'NONE',  ( -28.43739315969223824, -33.45000000000000995, -9.865911304835512041 ) ) ;
#7166=CARTESIAN_POINT ( 'NONE',  ( -22.97617564697422665, -34.74859572486943904, -7.102600956461224690 ) ) ;
#7167=CARTESIAN_POINT ( 'NONE',  ( -25.51477047955235378, -30.65140427513057730, 8.925456012876139766 ) ) ;
#7169=CARTESIAN_POINT ( 'NONE',  ( -39.37475178375516549, -31.70140427513057091, -1.538452329860249712 ) ) ;
#7177=CARTESIAN_POINT ( 'NONE',  ( -25.94249218456686279, -40.65000000000000568, 7.963307464738195840 ) ) ;
#7188=CARTESIAN_POINT ( 'NONE',  ( -25.94249218456686279, -31.65000000000000568, 7.963307464738194952 ) ) ;
#7194=CARTESIAN_POINT ( 'NONE',  ( -21.59636165304264921, -44.19859572486944899, 1.277368040863740228 ) ) ;
#7195=CARTESIAN_POINT ( 'NONE',  ( -34.53486167607238144, -36.15000000000001279, -8.900167166472096270 ) ) ;
#7196=CARTESIAN_POINT ( 'NONE',  ( -22.40239342223677355, -35.90140427513058086, -3.811716262761597473 ) ) ;
#7197=( GEOMETRIC_REPRESENTATION_CONTEXT ( 3 ) GLOBAL_UNCERTAINTY_ASSIGNED_CONTEXT ( ( #5551 ) ) GLOBAL_UNIT_ASSIGNED_CONTEXT ( ( #7150, #321, #3635 ) ) REPRESENTATION_CONTEXT ( 'NONE', 'WORKASPACE' ) );
#7200=CARTESIAN_POINT ( 'NONE',  ( -22.97617564697422665, -40.74859572486943904, -7.102600956461224690 ) ) ;
#7201=CARTESIAN_POINT ( 'NONE',  ( -25.46513832392765408, -37.65000000000000568, 8.900167166472096270 ) ) ;
#7206=ORIENTED_EDGE ( 'NONE', *, *, #4736, .T. ) ;
#7208=CARTESIAN_POINT ( 'NONE',  ( -23.95213185889994989, -47.49859572486944614, 5.972947139071243861 ) ) ;
#7209=CARTESIAN_POINT ( 'NONE',  ( -21.51138689804841420, -32.90140427513058086, -4.265706762501151772 ) ) ;
#7213=CARTESIAN_POINT ( 'NONE',  ( -20.12537475255788522, -36.05140427513057944, -1.507589171976365439 ) ) ;
#7220=CARTESIAN_POINT ( 'NONE',  ( -22.03669253526174998, -46.34999999999998721, 4.057507815433014642 ) ) ;
#7227=CARTESIAN_POINT ( 'NONE',  ( -21.61293655684001536, -33.20140427513057091, 1.382017864820032971 ) ) ;
#7231=CARTESIAN_POINT ( 'NONE',  ( -21.17260567462091103, -34.04999999999999005, -1.398121909749241887 ) ) ;
#7236=CARTESIAN_POINT ( 'NONE',  ( -37.54950433343896776, -45.39859572486944472, 3.906122232810848249 ) ) ;
#7237=CARTESIAN_POINT ( 'NONE',  ( -28.43739315969223824, -33.45000000000000995, -9.865911304835512041 ) ) ;
#7238=CARTESIAN_POINT ( 'NONE',  ( -36.35910488754074521, -43.25140427513058228, 6.280328284105565650 ) ) ;
#7242=CARTESIAN_POINT ( 'NONE',  ( -28.46154767013959486, -41.79859572486943620, 9.374751783755112200 ) ) ;
#7243=CARTESIAN_POINT ( 'NONE',  ( -20.61696076434619584, -37.20000000000000284, 1.486127417882100676 ) ) ;
#7249=CARTESIAN_POINT ( 'NONE',  ( -22.01140368885771892, -47.34859572486942625, 4.007875659808335378 ) ) ;
#7250=CARTESIAN_POINT ( 'NONE',  ( -31.56260684030781505, -49.95000000000000995, 9.865911304835510265 ) ) ;
#7254=CARTESIAN_POINT ( 'NONE',  ( -25.51477047955235378, -45.65140427513058086, 8.925456012876139766 ) ) ;
#7261=CARTESIAN_POINT ( 'NONE',  ( -28.67030704715798350, -40.80000000000000426, 8.395350895058669494 ) ) ;
#7267=CARTESIAN_POINT ( 'NONE',  ( -31.48612741788231517, -48.30000000000001137, -9.383039235653804155 ) ) ;
#7271=CARTESIAN_POINT ( 'NONE',  ( -37.59760657776328685, -37.40140427513058796, 3.811716262761598362 ) ) ;
#7274=CARTESIAN_POINT ( 'NONE',  ( -22.03669253526174998, -31.34999999999999432, 4.057507815433014642 ) ) ;
#7281=CARTESIAN_POINT ( 'NONE',  ( -28.51387258211773812, -34.80000000000000426, 9.383039235653802379 ) ) ;
#7282=CARTESIAN_POINT ( 'NONE',  ( -25.99212434019154472, -42.65140427513058086, 7.988596311142242890 ) ) ;
#7285=CARTESIAN_POINT ( 'NONE',  ( -25.73429323749904185, -34.59859572486944046, -8.488613101951701267 ) ) ;
#7286=CARTESIAN_POINT ( 'NONE',  ( -36.71751442127229836, -42.00000000000000711, -6.717514421272142044 ) ) ;
#7294=CARTESIAN_POINT ( 'NONE',  ( -23.95213185889994989, -50.49859572486944614, 5.972947139071243861 ) ) ;
#7295=CARTESIAN_POINT ( 'NONE',  ( -20.12537475255788522, -30.05140427513057944, -1.507589171976365439 ) ) ;
#7298=CARTESIAN_POINT ( 'NONE',  ( -38.87487832006816291, -49.85140427513058370, -4.584493831696867971 ) ) ;
#7306=CARTESIAN_POINT ( 'NONE',  ( -31.32969295284206979, -42.30000000000000426, -8.395350895058669494 ) ) ;
#7310=CARTESIAN_POINT ( 'NONE',  ( -34.31290974752564438, -47.10000000000000142, 8.464561979789547053 ) ) ;
#7314=CARTESIAN_POINT ( 'NONE',  ( -33.90612223281073057, -31.10140427513058370, 7.549504333439023718 ) ) ;
#7320=CARTESIAN_POINT ( 'NONE',  ( -28.67030704715798350, -34.80000000000000426, 8.395350895058669494 ) ) ;
#7322=CARTESIAN_POINT ( 'NONE',  ( -31.56260684030781505, -46.94999999999999574, 9.865911304835508489 ) ) ;
#7325=CARTESIAN_POINT ( 'NONE',  ( -38.46456197978948666, -47.40000000000001279, 4.312909747525784709 ) ) ;
#7326=CARTESIAN_POINT ( 'NONE',  ( -22.40239342223677355, -44.90140427513058086, -3.811716262761597473 ) ) ;
#7330=CARTESIAN_POINT ( 'NONE',  ( -20.14280263777121149, -35.04859572486943620, -1.617624508639600833 ) ) ;
#7337=CARTESIAN_POINT ( 'NONE',  ( -37.57355545560112375, -50.40000000000000568, 3.858919247786223305 ) ) ;
#7338=CARTESIAN_POINT ( 'NONE',  ( -20.60867331244750034, -32.19859572486942767, 1.433802505903951419 ) ) ;
#7339=CARTESIAN_POINT ( 'NONE',  ( -31.43380250590416125, -41.30140427513058654, -9.391326687552492558 ) ) ;
#7343=CARTESIAN_POINT ( 'NONE',  ( -25.51477047955235378, -48.65140427513057375, 8.925456012876139766 ) ) ;
#7351=CARTESIAN_POINT ( 'NONE',  ( -25.94249218456686279, -46.65000000000001279, 7.963307464738195840 ) ) ;
#7358=CARTESIAN_POINT ( 'NONE',  ( -21.53543802021056663, -42.90000000000000568, -4.312909747525783821 ) ) ;
#7362=CARTESIAN_POINT ( 'NONE',  ( -35.97294713907137975, -32.00140427513057517, -6.047868141099968398 ) ) ;
#7365=CARTESIAN_POINT ( 'NONE',  ( -36.01040764008574513, -36.00000000000000711, -6.010407640085605685 ) ) ;
#7371=CARTESIAN_POINT ( 'NONE',  ( -25.68709025247441602, -45.60000000000000853, -8.464561979789547053 ) ) ;
#7372=CARTESIAN_POINT ( 'NONE',  ( -36.31971658582311591, -32.25000000000000711, 6.319716585823199395 ) ) ;
#7373=SHAPE_REPRESENTATION ( 'shock absorber', ( #2554 ), #2987 ) ;
#7378=CARTESIAN_POINT ( 'NONE',  ( -39.39132668755255651, -45.69859572486943478, -1.433802505903950308 ) ) ;
#7384=CARTESIAN_POINT ( 'NONE',  ( -28.61798213517984024, -32.79859572486943620, 8.387063443159973986 ) ) ;
#7385=CARTESIAN_POINT ( 'NONE',  ( -25.41550616830297571, -41.64859572486943762, 8.874878320068054549 ) ) ;
#7386=CARTESIAN_POINT ( 'NONE',  ( -28.56619749409589204, -39.80140427513057944, 9.391326687552490782 ) ) ;
#7389=CARTESIAN_POINT ( 'NONE',  ( -21.51138689804841420, -41.90140427513058086, -4.265706762501151772 ) ) ;
#7396=CARTESIAN_POINT ( 'NONE',  ( -36.04786814110010340, -33.99859572486943904, -5.972947139071243861 ) ) ;
#7397=CARTESIAN_POINT ( 'NONE',  ( -25.46513832392765408, -37.65000000000000568, 8.900167166472096270 ) ) ;
#7402=CARTESIAN_POINT ( 'NONE',  ( -39.86591130483550671, -41.55000000000001137, 1.562606840307984468 ) ) ;
#7406=CARTESIAN_POINT ( 'NONE',  ( -37.93801861833426159, -46.85140427513056949, -4.107139971057695682 ) ) ;
#7408=CARTESIAN_POINT ( 'NONE',  ( -33.85891924778610473, -41.10000000000000142, 7.573555455601171715 ) ) ;
#7415=CARTESIAN_POINT ( 'NONE',  ( -36.71751442127229836, -48.00000000000000711, -6.717514421272142044 ) ) ;
#7416=CARTESIAN_POINT ( 'NONE',  ( -37.93801861833426159, -46.85140427513056949, -4.107139971057695682 ) ) ;
#7422=CARTESIAN_POINT ( 'NONE',  ( -36.75497492228666374, -42.99859572486943904, -6.680053920257780220 ) ) ;
#7424=CARTESIAN_POINT ( 'NONE',  ( -23.28248557872775137, -31.50000000000000711, 6.717514421272141156 ) ) ;
#7427=CARTESIAN_POINT ( 'NONE',  ( -31.39812190974910422, -46.94999999999998863, 8.827394325379140483 ) ) ;
#7428=CARTESIAN_POINT ( 'NONE',  ( -37.02382435302582309, -39.24859572486943904, 7.102600956461226467 ) ) ;
#7429=CARTESIAN_POINT ( 'NONE',  ( -25.51477047955235378, -45.65140427513058086, 8.925456012876139766 ) ) ;
#7433=CARTESIAN_POINT ( 'NONE',  ( -36.68005392025794009, -41.00140427513057517, -6.754974922286504757 ) ) ;
#7440=CARTESIAN_POINT ( 'NONE',  ( -38.39535089505872634, -50.70000000000000995, -1.329692952841885267 ) ) ;
#7441=CARTESIAN_POINT ( 'NONE',  ( -31.48612741788231517, -33.30000000000000426, -9.383039235653804155 ) ) ;
#7446=CARTESIAN_POINT ( 'NONE',  ( -28.43739315969223824, -45.45000000000000995, -9.865911304835512041 ) ) ;
#7451=CARTESIAN_POINT ( 'NONE',  ( -37.93801861833426159, -43.85140427513058370, -4.107139971057695682 ) ) ;
#7453=CARTESIAN_POINT ( 'NONE',  ( -38.82739432537914581, -44.55000000000000426, 1.398121909749243663 ) ) ;
#7459=CARTESIAN_POINT ( 'NONE',  ( -28.43739315969223824, -48.44999999999999574, -9.865911304835512041 ) ) ;
#7460=CARTESIAN_POINT ( 'NONE',  ( -28.54686042191934092, -47.45140427513057091, -8.818680382772479120 ) ) ;
#7464=CARTESIAN_POINT ( 'NONE',  ( -25.41550616830297571, -50.64859572486944472, 8.874878320068054549 ) ) ;
#7468=CARTESIAN_POINT ( 'NONE',  ( -31.39812190974910422, -49.95000000000000995, 8.827394325379140483 ) ) ;
#7469=CARTESIAN_POINT ( 'NONE',  ( -37.02382435302582309, -36.24859572486943904, 7.102600956461226467 ) ) ;
#7470=CARTESIAN_POINT ( 'NONE',  ( -34.36011273255026310, -37.10140427513057659, 8.440510857627391061 ) ) ;
#7481=CARTESIAN_POINT ( 'NONE',  ( -22.45049566656107842, -34.89859572486943762, -3.906122232810846917 ) ) ;
#7482=CARTESIAN_POINT ( 'NONE',  ( -31.48612741788231517, -39.30000000000001137, -9.383039235653804155 ) ) ;
#7488=CARTESIAN_POINT ( 'NONE',  ( -38.90016716647221529, -50.84999999999999432, -4.534861676072185155 ) ) ;
#7493=CARTESIAN_POINT ( 'NONE',  ( -28.54686042191934092, -44.45140427513058512, -8.818680382772479120 ) ) ;
#7496=CARTESIAN_POINT ( 'NONE',  ( -25.94249218456686279, -43.64999999999999858, 7.963307464738194952 ) ) ;
#7501=CARTESIAN_POINT ( 'NONE',  ( -39.86591130483550671, -50.55000000000001137, 1.562606840307984468 ) ) ;
#7502=CARTESIAN_POINT ( 'NONE',  ( -31.27736804086391942, -47.30140427513057944, -8.403638346957361449 ) ) ;
#7505=CARTESIAN_POINT ( 'NONE',  ( -22.97617564697422665, -49.74859572486944614, -7.102600956461224690 ) ) ;
#7512=CARTESIAN_POINT ( 'NONE',  ( -22.45049566656107842, -31.89859572486943762, -3.906122232810846917 ) ) ;
#7513=CARTESIAN_POINT ( 'NONE',  ( -22.97617564697422665, -43.74859572486943904, -7.102600956461224690 ) ) ;
#7514=CARTESIAN_POINT ( 'NONE',  ( -39.37475178375516549, -37.70140427513057091, -1.538452329860249712 ) ) ;
#7518=CARTESIAN_POINT ( 'NONE',  ( -20.13408869516453947, -31.05000000000000782, -1.562606840307983136 ) ) ;
#7525=CARTESIAN_POINT ( 'NONE',  ( -33.81171626276147890, -36.09859572486943335, 7.597606577763319713 ) ) ;
#7526=CARTESIAN_POINT ( 'NONE',  ( -38.46456197978948666, -35.40000000000000568, 4.312909747525784709 ) ) ;
#7528=CARTESIAN_POINT ( 'NONE',  ( -21.09983283352784156, -49.35000000000000853, 4.534861676072186043 ) ) ;
#7533=CARTESIAN_POINT ( 'NONE',  ( -24.02705286092866643, -42.50140427513057517, 6.047868141099968398 ) ) ;
#7537=CARTESIAN_POINT ( 'NONE',  ( -21.17260567462091103, -46.05000000000000426, -1.398121909749241887 ) ) ;
#7542=CARTESIAN_POINT ( 'NONE',  ( -31.32969295284206979, -39.30000000000001137, -8.395350895058669494 ) ) ;
#7546=CARTESIAN_POINT ( 'NONE',  ( -38.92545601287626056, -51.84859572486944757, -4.485229520447501450 ) ) ;
#7548=CARTESIAN_POINT ( 'NONE',  ( -38.90016716647221529, -32.85000000000000142, -4.534861676072185155 ) ) ;
#7553=CARTESIAN_POINT ( 'NONE',  ( -33.81171626276147890, -42.09859572486944046, 7.597606577763319713 ) ) ;
#7554=CARTESIAN_POINT ( 'NONE',  ( -34.58449383169706692, -46.14859572486944472, -8.874878320068054549 ) ) ;
#7555=CARTESIAN_POINT ( 'NONE',  ( -31.43380250590416125, -47.30140427513057944, -9.391326687552492558 ) ) ;
#7566=CARTESIAN_POINT ( 'NONE',  ( -21.17260567462091458, -49.04999999999999716, -1.398121909749242331 ) ) ;
#7567=CARTESIAN_POINT ( 'NONE',  ( -37.06321265474346660, -35.24999999999998579, 7.063212654743582952 ) ) ;
#7569=CARTESIAN_POINT ( 'NONE',  ( -38.46456197978948666, -50.40000000000000568, 4.312909747525784709 ) ) ;
#7577=CARTESIAN_POINT ( 'NONE',  ( -31.45313957808072303, -45.95140427513058512, 8.818680382772479120 ) ) ;
#7582=CARTESIAN_POINT ( 'NONE',  ( -36.31971658582311591, -47.25000000000000711, 6.319716585823200283 ) ) ;
#7587=CARTESIAN_POINT ( 'NONE',  ( -22.42644454439892598, -39.90000000000000568, -3.858919247786222861 ) ) ;
#7590=CARTESIAN_POINT ( 'NONE',  ( -34.31290974752564438, -32.10000000000000142, 8.464561979789547053 ) ) ;
#7596=CARTESIAN_POINT ( 'NONE',  ( -23.95213185889994989, -35.49859572486943193, 5.972947139071243861 ) ) ;
#7597=CARTESIAN_POINT ( 'NONE',  ( -38.44051085762733777, -51.39859572486944472, 4.360112732550414982 ) ) ;
#7598=CARTESIAN_POINT ( 'NONE',  ( -37.10260095646111012, -46.25140427513058228, 7.023824353025939438 ) ) ;
#7601=CARTESIAN_POINT ( 'NONE',  ( -21.09983283352784156, -31.34999999999999787, 4.534861676072186043 ) ) ;
#7610=CARTESIAN_POINT ( 'NONE',  ( -23.71967171589458445, -37.74859572486943904, -6.359104887540838469 ) ) ;
#7611=CARTESIAN_POINT ( 'NONE',  ( -25.46513832392765408, -40.65000000000000568, 8.900167166472096270 ) ) ;
#7614=CARTESIAN_POINT ( 'NONE',  ( -31.48612741788231517, -45.30000000000000426, -9.383039235653804155 ) ) ;
#7619=CARTESIAN_POINT ( 'NONE',  ( -37.59760657776328685, -49.40140427513058086, 3.811716262761598362 ) ) ;
#7629=CARTESIAN_POINT ( 'NONE',  ( -36.01040764008574513, -39.00000000000000711, -6.010407640085605685 ) ) ;
#7633=CARTESIAN_POINT ( 'NONE',  ( -20.61696076434619584, -34.20000000000000995, 1.486127417882100676 ) ) ;
#7635=CARTESIAN_POINT ( 'NONE',  ( -36.71751442127229836, -36.00000000000000711, -6.717514421272142044 ) ) ;
#7642=CARTESIAN_POINT ( 'NONE',  ( -28.61798213517984024, -35.79859572486943620, 8.387063443159973986 ) ) ;
#7643=CARTESIAN_POINT ( 'NONE',  ( -34.58449383169706692, -49.14859572486945183, -8.874878320068054549 ) ) ;
#7644=CARTESIAN_POINT ( 'NONE',  ( -24.02705286092866643, -33.50140427513058228, 6.047868141099968398 ) ) ;
#7655=CARTESIAN_POINT ( 'NONE',  ( -22.45049566656107842, -40.89859572486943762, -3.906122232810846917 ) ) ;
#7657=CARTESIAN_POINT ( 'NONE',  ( -20.61696076434619584, -40.20000000000000995, 1.486127417882100676 ) ) ;
#7659=CARTESIAN_POINT ( 'NONE',  ( -34.53486167607238144, -48.15000000000001279, -8.900167166472096270 ) ) ;
#7667=CARTESIAN_POINT ( 'NONE',  ( -31.39812190974910422, -31.95000000000000639, 8.827394325379140483 ) ) ;
#7675=CARTESIAN_POINT ( 'NONE',  ( -23.68028341417693738, -39.74999999999999289, -6.319716585823198507 ) ) ;
#7680=CARTESIAN_POINT ( 'NONE',  ( -31.48612741788231517, -33.30000000000000426, -9.383039235653804155 ) ) ;
#7683=CARTESIAN_POINT ( 'NONE',  ( -21.09983283352783801, -37.35000000000000853, 4.534861676072186043 ) ) ;
#7689=CARTESIAN_POINT ( 'NONE',  ( -31.38201786482021305, -43.29859572486943620, -8.387063443159975762 ) ) ;
#7691=CARTESIAN_POINT ( 'NONE',  ( -34.26570676250101855, -45.09859572486944046, 8.488613101951703044 ) ) ;
#7692=CARTESIAN_POINT ( 'NONE',  ( -28.54686042191934092, -32.45140427513058512, -8.818680382772479120 ) ) ;
#7705=CARTESIAN_POINT ( 'NONE',  ( -37.98859631114233792, -42.84859572486944046, -4.007875659808334490 ) ) ;
#7706=CARTESIAN_POINT ( 'NONE',  ( -22.93678734525658314, -45.74999999999999289, -7.063212654743582952 ) ) ;
#7709=CARTESIAN_POINT ( 'NONE',  ( -31.61762450863942320, -30.95140427513058157, 9.857197362228843573 ) ) ;
#7717=CARTESIAN_POINT ( 'NONE',  ( -28.67030704715798350, -31.80000000000000782, 8.395350895058669494 ) ) ;
#7725=CARTESIAN_POINT ( 'NONE',  ( -21.60464910494133406, -34.20000000000000995, 1.329692952841886155 ) ) ;
#7729=CARTESIAN_POINT ( 'NONE',  ( -36.71751442127229836, -30.00000000000000711, -6.717514421272142044 ) ) ;
#7731=CARTESIAN_POINT ( 'NONE',  ( -28.51387258211773812, -40.80000000000000426, 9.383039235653802379 ) ) ;
#7734=CARTESIAN_POINT ( 'NONE',  ( -38.40363834695740053, -42.69859572486944188, -1.277368040863739118 ) ) ;
#7735=CARTESIAN_POINT ( 'NONE',  ( -20.14280263777121149, -47.04859572486944330, -1.617624508639600833 ) ) ;
#7736=CARTESIAN_POINT ( 'NONE',  ( -37.93801861833426159, -31.85140427513056594, -4.107139971057695682 ) ) ;
#7740=CARTESIAN_POINT ( 'NONE',  ( -31.56260684030781505, -40.95000000000000995, 9.865911304835510265 ) ) ;
#7746=CARTESIAN_POINT ( 'NONE',  ( -31.34310424141748896, -44.94859572486942767, 8.836108267985801845 ) ) ;
#7747=CARTESIAN_POINT ( 'NONE',  ( -36.71751442127229836, -48.00000000000000711, -6.717514421272142044 ) ) ;
#7749=CARTESIAN_POINT ( 'NONE',  ( -37.10260095646111012, -40.25140427513058228, 7.023824353025939438 ) ) ;
#7758=CARTESIAN_POINT ( 'NONE',  ( -36.31971658582311591, -35.24999999999998579, 6.319716585823199395 ) ) ;
#7765=CARTESIAN_POINT ( 'NONE',  ( -37.96330746473829976, -44.85000000000001563, -4.057507815433013754 ) ) ;
#7768=CARTESIAN_POINT ( 'NONE',  ( -21.53543802021056663, -36.90000000000000568, -4.312909747525783821 ) ) ;
#7770=CARTESIAN_POINT ( 'NONE',  ( -37.06321265474346660, -38.25000000000001421, 7.063212654743582952 ) ) ;
#7772=CARTESIAN_POINT ( 'NONE',  ( -20.61696076434619584, -40.20000000000000995, 1.486127417882100676 ) ) ;
#7775=CARTESIAN_POINT ( 'NONE',  ( -28.65689575858256077, -49.44859572486943478, -8.836108267985801845 ) ) ;
#7776=CARTESIAN_POINT ( 'NONE',  ( -23.28248557872775137, -37.50000000000000711, 6.717514421272141156 ) ) ;
#7778=CARTESIAN_POINT ( 'NONE',  ( -22.06198138166579170, -39.35140427513057659, 4.107139971057695682 ) ) ;
#7781=CARTESIAN_POINT ( 'NONE',  ( -37.06321265474346660, -41.25000000000000711, 7.063212654743582952 ) ) ;
#7787=CARTESIAN_POINT ( 'NONE',  ( 0.000000000000000000, 0.000000000000000000, 0.000000000000000000 ) ) ;
#7790=CARTESIAN_POINT ( 'NONE',  ( -28.61798213517984024, -41.79859572486943620, 8.387063443159973986 ) ) ;
#7791=CARTESIAN_POINT ( 'NONE',  ( -22.93678734525658314, -48.75000000000001421, -7.063212654743582952 ) ) ;
#7792=EDGE_CURVE ( 'NONE', #282, #7915, #676, .T. ) ;
#7795=CARTESIAN_POINT ( 'NONE',  ( -34.48522952044771017, -32.15140427513058086, -8.925456012876139766 ) ) ;
#7803=CARTESIAN_POINT ( 'NONE',  ( -28.60187809025093841, -36.45000000000000284, -8.827394325379140483 ) ) ;
#7808=ADVANCED_BREP_SHAPE_REPRESENTATION ( '', ( #5903, #2554 ), #2987 ) ;
#7817=CARTESIAN_POINT ( 'NONE',  ( -28.51387258211773812, -37.80000000000000426, 9.383039235653802379 ) ) ;
#7820=CARTESIAN_POINT ( 'NONE',  ( -33.81171626276147890, -51.09859572486944046, 7.597606577763319713 ) ) ;
#7821=CARTESIAN_POINT ( 'NONE',  ( -20.61696076434619584, -40.20000000000000995, 1.486127417882100676 ) ) ;
#7822=CARTESIAN_POINT ( 'NONE',  ( -35.97294713907137975, -38.00140427513057517, -6.047868141099968398 ) ) ;
#7826=CARTESIAN_POINT ( 'NONE',  ( -38.46456197978948666, -38.40000000000000568, 4.312909747525784709 ) ) ;
#7833=CARTESIAN_POINT ( 'NONE',  ( -36.75497492228666374, -33.99859572486943904, -6.680053920257780220 ) ) ;
#7834=CARTESIAN_POINT ( 'NONE',  ( -21.12512167993187973, -30.35140427513058015, 4.584493831696868860 ) ) ;
#7836=CARTESIAN_POINT ( 'NONE',  ( -20.62524821624488069, -33.20140427513057091, 1.538452329860250378 ) ) ;
#7843=CARTESIAN_POINT ( 'NONE',  ( -23.98959235991431171, -40.50000000000000711, 6.010407640085604797 ) ) ;
#7850=PLANE ( 'NONE',  #5426 ) ;
#7857=CARTESIAN_POINT ( 'NONE',  ( -38.46456197978948666, -47.40000000000001279, 4.312909747525784709 ) ) ;
#7861=CARTESIAN_POINT ( 'NONE',  ( -23.95213185889994989, -50.49859572486944614, 5.972947139071243861 ) ) ;
#7862=CARTESIAN_POINT ( 'NONE',  ( -31.56260684030781505, -37.94999999999998153, 9.865911304835510265 ) ) ;
#7863=CARTESIAN_POINT ( 'NONE',  ( -21.16389173201424612, -36.05140427513057944, -1.343104241417630185 ) ) ;
#7867=CARTESIAN_POINT ( 'NONE',  ( -21.07454398712378918, -35.34859572486944046, 4.485229520447505003 ) ) ;
#7868=CARTESIAN_POINT ( 'NONE',  ( -21.53543802021056663, -36.90000000000000568, -4.312909747525783821 ) ) ;
#7875=CARTESIAN_POINT ( 'NONE',  ( -37.54950433343896776, -51.39859572486944472, 3.906122232810848249 ) ) ;
#7876=CARTESIAN_POINT ( 'NONE',  ( -38.87487832006816291, -34.85140427513057659, -4.584493831696867971 ) ) ;
#7879=CARTESIAN_POINT ( 'NONE',  ( -38.87487832006816291, -31.85140427513056594, -4.584493831696867971 ) ) ;
#7887=CARTESIAN_POINT ( 'NONE',  ( -37.96330746473829976, -44.85000000000001563, -4.057507815433013754 ) ) ;
#7892=CARTESIAN_POINT ( 'NONE',  ( -24.02705286092866643, -36.50140427513057517, 6.047868141099968398 ) ) ;
#7896=CARTESIAN_POINT ( 'NONE',  ( -25.94249218456686279, -37.65000000000000568, 7.963307464738194952 ) ) ;
#7898=CARTESIAN_POINT ( 'NONE',  ( -36.71751442127229836, -48.00000000000000711, -6.717514421272142044 ) ) ;
#7902=CARTESIAN_POINT ( 'NONE',  ( -34.10713997105786888, -46.14859572486944472, -7.938018618334151455 ) ) ;
#7903=CARTESIAN_POINT ( 'NONE',  ( -38.46456197978948666, -38.40000000000000568, 4.312909747525784709 ) ) ;
#7904=CARTESIAN_POINT ( 'NONE',  ( -31.27736804086391942, -41.30140427513058654, -8.403638346957361449 ) ) ;
#7908=CARTESIAN_POINT ( 'NONE',  ( -25.41550616830297571, -38.64859572486943762, 8.874878320068054549 ) ) ;
#7909=CARTESIAN_POINT ( 'NONE',  ( -25.46513832392765408, -40.65000000000000568, 8.900167166472096270 ) ) ;
#7910=AXIS2_PLACEMENT_3D ( 'NONE', #4576, #1968, #8105 ) ;
#7915=VERTEX_POINT ( 'NONE', #4109 ) ;
#7918=CARTESIAN_POINT ( 'NONE',  ( -33.81171626276147890, -51.09859572486944046, 7.597606577763319713 ) ) ;
#7919=CARTESIAN_POINT ( 'NONE',  ( -34.36011273255026310, -31.10140427513058370, 8.440510857627391061 ) ) ;
#7922=CARTESIAN_POINT ( 'NONE',  ( -38.87487832006816291, -37.85140427513057659, -4.584493831696867971 ) ) ;
#7928=CARTESIAN_POINT ( 'NONE',  ( -26.14108075221394856, -39.60000000000000853, -7.573555455601170827 ) ) ;
#7932=CARTESIAN_POINT ( 'NONE',  ( -22.93678734525658314, -45.74999999999999289, -7.063212654743582952 ) ) ;
#7935=CARTESIAN_POINT ( 'NONE',  ( -36.35910488754074521, -37.25140427513058228, 6.280328284105565650 ) ) ;
#7940=CARTESIAN_POINT ( 'NONE',  ( -37.57355545560112375, -32.40000000000000568, 3.858919247786223305 ) ) ;
#7943=CARTESIAN_POINT ( 'NONE',  ( -34.31290974752564438, -47.10000000000000142, 8.464561979789547053 ) ) ;
#7945=CARTESIAN_POINT ( 'NONE',  ( -38.81868038277247734, -51.54859572486944330, 1.453139578080855365 ) ) ;
#7946=CARTESIAN_POINT ( 'NONE',  ( -25.68709025247441602, -39.60000000000000853, -8.464561979789547053 ) ) ;
#7947=CARTESIAN_POINT ( 'NONE',  ( -24.02705286092866643, -42.50140427513057517, 6.047868141099968398 ) ) ;
#7951=CARTESIAN_POINT ( 'NONE',  ( -34.26570676250101855, -36.09859572486943335, 8.488613101951703044 ) ) ;
#7952=CARTESIAN_POINT ( 'NONE',  ( -38.90016716647221529, -41.84999999999999432, -4.534861676072185155 ) ) ;
#7959=CARTESIAN_POINT ( 'NONE',  ( -36.28032828410546529, -48.24859572486943904, 6.359104887540839357 ) ) ;
#7960=CARTESIAN_POINT ( 'NONE',  ( -34.48522952044771017, -32.15140427513058086, -8.925456012876139766 ) ) ;
#7964=CARTESIAN_POINT ( 'NONE',  ( -20.62524821624488069, -45.20140427513059223, 1.538452329860250378 ) ) ;
#7974=CARTESIAN_POINT ( 'NONE',  ( -36.31971658582311591, -38.25000000000001421, 6.319716585823199395 ) ) ;
#7979=CARTESIAN_POINT ( 'NONE',  ( -34.53486167607238144, -45.14999999999999858, -8.900167166472096270 ) ) ;
#7983=CARTESIAN_POINT ( 'NONE',  ( -37.59760657776328685, -31.40140427513058086, 3.811716262761598362 ) ) ;
#7987=CARTESIAN_POINT ( 'NONE',  ( -31.32969295284206979, -33.30000000000000426, -8.395350895058669494 ) ) ;
#7989=CARTESIAN_POINT ( 'NONE',  ( -38.90016716647221529, -47.85000000000000142, -4.534861676072185155 ) ) ;
#7994=CARTESIAN_POINT ( 'NONE',  ( -39.86591130483550671, -41.55000000000001137, 1.562606840307984468 ) ) ;
#7995=CARTESIAN_POINT ( 'NONE',  ( -33.85891924778610473, -32.10000000000000142, 7.573555455601171715 ) ) ;
#7999=CARTESIAN_POINT ( 'NONE',  ( -34.58449383169706692, -37.14859572486943762, -8.874878320068054549 ) ) ;
#8005=CARTESIAN_POINT ( 'NONE',  ( -38.82739432537914581, -47.54999999999999716, 1.398121909749243441 ) ) ;
#8006=CARTESIAN_POINT ( 'NONE',  ( -25.73429323749904185, -31.59859572486943335, -8.488613101951701267 ) ) ;
#8007=CARTESIAN_POINT ( 'NONE',  ( -31.43380250590416125, -29.30140427513058299, -9.391326687552492558 ) ) ;
#8011=CARTESIAN_POINT ( 'NONE',  ( -21.51138689804841420, -47.90140427513058086, -4.265706762501151772 ) ) ;
#8017=CARTESIAN_POINT ( 'NONE',  ( -21.17260567462091458, -46.05000000000001137, -1.398121909749242331 ) ) ;
#8022=CARTESIAN_POINT ( 'NONE',  ( -23.28248557872775137, -46.50000000000000711, 6.717514421272141156 ) ) ;
#8026=CARTESIAN_POINT ( 'NONE',  ( -31.45313957808072303, -33.95140427513058512, 8.818680382772479120 ) ) ;
#8030=CARTESIAN_POINT ( 'NONE',  ( -37.96330746473829976, -38.85000000000000853, -4.057507815433013754 ) ) ;
#8036=CARTESIAN_POINT ( 'NONE',  ( -34.31290974752564438, -44.10000000000000853, 8.464561979789547053 ) ) ;
#8037=CARTESIAN_POINT ( 'NONE',  ( -34.05750781543318340, -30.15000000000000213, -7.963307464738195840 ) ) ;
#8040=CARTESIAN_POINT ( 'NONE',  ( -31.53845232986046554, -34.29859572486943620, -9.374751783755117529 ) ) ;
#8047=CARTESIAN_POINT ( 'NONE',  ( -22.03669253526174998, -49.35000000000000853, 4.057507815433014642 ) ) ;
#8048=CARTESIAN_POINT ( 'NONE',  ( -20.60867331244750034, -35.19859572486944188, 1.433802505903951419 ) ) ;
#8049=CARTESIAN_POINT ( 'NONE',  ( -22.89739904353894318, -41.75140427513057517, -7.023824353025938549 ) ) ;
#8052=CARTESIAN_POINT ( 'NONE',  ( -25.51477047955235378, -42.65140427513058086, 8.925456012876139766 ) ) ;
#8059=CARTESIAN_POINT ( 'NONE',  ( -28.61798213517984024, -32.79859572486943620, 8.387063443159973986 ) ) ;
#8061=CARTESIAN_POINT ( 'NONE',  ( -20.61696076434619584, -37.20000000000000284, 1.486127417882100676 ) ) ;
#8067=CARTESIAN_POINT ( 'NONE',  ( -37.06321265474346660, -41.25000000000000711, 7.063212654743582952 ) ) ;
#8072=CARTESIAN_POINT ( 'NONE',  ( -28.54686042191934092, -29.45140427513057801, -8.818680382772479120 ) ) ;
#8076=CARTESIAN_POINT ( 'NONE',  ( -33.85891924778610473, -38.10000000000000853, 7.573555455601171715 ) ) ;
#8082=ORIENTED_EDGE ( 'NONE', *, *, #4137, .T. ) ;
#8084=CARTESIAN_POINT ( 'NONE',  ( -25.68709025247441602, -42.60000000000000853, -8.464561979789547053 ) ) ;
#8085=CARTESIAN_POINT ( 'NONE',  ( -21.16389173201424612, -45.05140427513057944, -1.343104241417630185 ) ) ;
#8090=CARTESIAN_POINT ( 'NONE',  ( -21.07454398712378918, -47.34859572486942625, 4.485229520447505003 ) ) ;
#8092=CARTESIAN_POINT ( 'NONE',  ( -34.53486167607238855, -30.15000000000000568, -8.900167166472096270 ) ) ;
#8097=CARTESIAN_POINT ( 'NONE',  ( -28.60187809025093841, -45.45000000000000995, -8.827394325379140483 ) ) ;
#8098=CARTESIAN_POINT ( 'NONE',  ( -34.26570676250101855, -36.09859572486943335, 8.488613101951703044 ) ) ;
#8099=CARTESIAN_POINT ( 'NONE',  ( -38.48861310195163554, -43.40140427513058796, 4.265706762501153548 ) ) ;
#8103=CARTESIAN_POINT ( 'NONE',  ( -39.37475178375516549, -49.70140427513058512, -1.538452329860249712 ) ) ;
#8105=DIRECTION ( 'NONE',  ( -0.7071067811865587860, 0.000000000000000000, -0.7071067811865362485 ) ) ;
#8110=CARTESIAN_POINT ( 'NONE',  ( -21.18131961722757595, -35.04859572486943620, -1.453139578080854699 ) ) ;
#8111=CARTESIAN_POINT ( 'NONE',  ( -37.06321265474346660, -38.25000000000001421, 7.063212654743582952 ) ) ;
#8117=CARTESIAN_POINT ( 'NONE',  ( -21.09983283352784156, -43.35000000000000853, 4.534861676072186043 ) ) ;
#8121=CARTESIAN_POINT ( 'NONE',  ( -31.45313957808072303, -42.95140427513058512, 8.818680382772479120 ) ) ;
#8124=CARTESIAN_POINT ( 'NONE',  ( -26.14108075221394856, -45.60000000000000853, -7.573555455601170827 ) ) ;
#8131=CARTESIAN_POINT ( 'NONE',  ( -21.53543802021056663, -45.90000000000001279, -4.312909747525783821 ) ) ;
#8132=CARTESIAN_POINT ( 'NONE',  ( -37.57355545560112375, -32.40000000000000568, 3.858919247786223305 ) ) ;
#8137=CARTESIAN_POINT ( 'NONE',  ( -22.97617564697422665, -46.74859572486943904, -7.102600956461224690 ) ) ;
#8143=CARTESIAN_POINT ( 'NONE',  ( -37.98859631114233792, -33.84859572486942625, -4.007875659808334490 ) ) ;
#8144=CARTESIAN_POINT ( 'NONE',  ( -25.41550616830297571, -38.64859572486943762, 8.874878320068054549 ) ) ;
#8145=CARTESIAN_POINT ( 'NONE',  ( -28.56619749409589204, -42.80140427513057944, 9.391326687552490782 ) ) ;
#8148=APPLICATION_CONTEXT ( 'automotive_design' ) ;
#8150=CARTESIAN_POINT ( 'NONE',  ( -39.87462524744216807, -46.55140427513058654, 1.507589171976367215 ) ) ;
#8154=DIRECTION ( 'NONE',  ( -0.7071067811865587860, 0.000000000000000000, -0.7071067811865362485 ) ) ;
#8157=CARTESIAN_POINT ( 'NONE',  ( -31.39812190974910422, -49.95000000000000995, 8.827394325379140483 ) ) ;
#8158=CARTESIAN_POINT ( 'NONE',  ( -38.46456197978948666, -32.40000000000000568, 4.312909747525784709 ) ) ;
#8166=CARTESIAN_POINT ( 'NONE',  ( -38.38706344316003793, -43.70140427513058512, -1.382017864820032083 ) ) ;
#8168=CARTESIAN_POINT ( 'NONE',  ( -34.05750781543319050, -42.15000000000000568, -7.963307464738194952 ) ) ;
#8174=CARTESIAN_POINT ( 'NONE',  ( -37.06321265474346660, -50.24999999999998579, 7.063212654743582952 ) ) ;
#8175=CARTESIAN_POINT ( 'NONE',  ( -31.32969295284206979, -33.30000000000000426, -8.395350895058669494 ) ) ;
#8179=CARTESIAN_POINT ( 'NONE',  ( -38.44051085762733777, -48.39859572486944472, 4.360112732550414982 ) ) ;
#8187=CARTESIAN_POINT ( 'NONE',  ( -33.85891924778610473, -47.10000000000000142, 7.573555455601171715 ) ) ;
#8188=CARTESIAN_POINT ( 'NONE',  ( -25.73429323749904185, -43.59859572486944046, -8.488613101951701267 ) ) ;
#8189=CARTESIAN_POINT ( 'NONE',  ( -28.38237549136062654, -38.45140427513057801, -9.857197362228843573 ) ) ;
#8202=CARTESIAN_POINT ( 'NONE',  ( -25.89286002894218086, -35.64859572486943051, 7.938018618334153231 ) ) ;
#8203=CARTESIAN_POINT ( 'NONE',  ( -28.43739315969223824, -33.45000000000000995, -9.865911304835512041 ) ) ;
#8205=CARTESIAN_POINT ( 'NONE',  ( -38.90016716647221529, -47.85000000000000853, -4.534861676072185155 ) ) ;
#8212=CARTESIAN_POINT ( 'NONE',  ( -21.61293655684001536, -42.20140427513058512, 1.382017864820032971 ) ) ;
#8217=CARTESIAN_POINT ( 'NONE',  ( -37.57355545560112375, -44.40000000000000568, 3.858919247786223305 ) ) ;
#8219=SHAPE_DEFINITION_REPRESENTATION ( #5076, #7373 ) ;
#8223=CARTESIAN_POINT ( 'NONE',  ( -37.57355545560112375, -35.40000000000000568, 3.858919247786223305 ) ) ;
#8227=CARTESIAN_POINT ( 'NONE',  ( -28.49241082802385350, -43.44859572486944188, -9.874625247442173404 ) ) ;
#8231=CARTESIAN_POINT ( 'NONE',  ( -28.65689575858256077, -40.44859572486944188, -8.836108267985801845 ) ) ;
#8232=CARTESIAN_POINT ( 'NONE',  ( -22.97617564697422665, -37.74859572486943904, -7.102600956461224690 ) ) ;
#8233=CARTESIAN_POINT ( 'NONE',  ( -34.48522952044771017, -44.15140427513058086, -8.925456012876139766 ) ) ;
#8245=CARTESIAN_POINT ( 'NONE',  ( -31.32969295284206979, -48.30000000000001137, -8.395350895058669494 ) ) ;
#8246=CARTESIAN_POINT ( 'NONE',  ( -39.38303923565386100, -32.70000000000000995, -1.486127417882099788 ) ) ;
#8248=CARTESIAN_POINT ( 'NONE',  ( -22.93678734525658314, -45.74999999999999289, -7.063212654743582952 ) ) ;
#8255=CARTESIAN_POINT ( 'NONE',  ( -22.06198138166579170, -45.35140427513057659, 4.107139971057695682 ) ) ;
#8259=CARTESIAN_POINT ( 'NONE',  ( -21.60464910494133406, -46.20000000000000284, 1.329692952841886155 ) ) ;
#8263=CARTESIAN_POINT ( 'NONE',  ( -26.14108075221394856, -42.60000000000000853, -7.573555455601170827 ) ) ;
#8265=CIRCLE ( 'NONE', #496, 0.5000000000000001110 ) ;
#8267=CARTESIAN_POINT ( 'NONE',  ( -25.41550616830297571, -47.64859572486945183, 8.874878320068054549 ) ) ;
#8273=CARTESIAN_POINT ( 'NONE',  ( -22.45049566656107842, -43.89859572486944472, -3.906122232810846917 ) ) ;
#8274=CARTESIAN_POINT ( 'NONE',  ( -39.39132668755255651, -45.69859572486943478, -1.433802505903950308 ) ) ;
#8275=CARTESIAN_POINT ( 'NONE',  ( -21.16389173201424612, -30.05140427513057944, -1.343104241417630185 ) ) ;
#8281=CARTESIAN_POINT ( 'NONE',  ( -36.71751442127229836, -30.00000000000000711, -6.717514421272142044 ) ) ;
#8288=CARTESIAN_POINT ( 'NONE',  ( -31.34310424141748896, -41.94859572486944188, 8.836108267985801845 ) ) ;
#8289=CARTESIAN_POINT ( 'NONE',  ( -31.56260684030781505, -43.95000000000000284, 9.865911304835510265 ) ) ;
#8291=CARTESIAN_POINT ( 'NONE',  ( -34.31290974752564438, -50.10000000000000853, 8.464561979789547053 ) ) ;
#8298=CARTESIAN_POINT ( 'NONE',  ( -26.09387776718931917, -47.60140427513058370, -7.549504333439021941 ) ) ;
#8306=CARTESIAN_POINT ( 'NONE',  ( -21.17260567462091458, -43.04999999999999005, -1.398121909749242331 ) ) ;
#8309=CARTESIAN_POINT ( 'NONE',  ( -36.75497492228666374, -51.99859572486943193, -6.680053920257780220 ) ) ;
#8311=CARTESIAN_POINT ( 'NONE',  ( -28.43739315969223824, -39.45000000000000284, -9.865911304835512041 ) ) ;
#8316=CARTESIAN_POINT ( 'NONE',  ( -31.34310424141748896, -41.94859572486944188, 8.836108267985801845 ) ) ;
#8317=CARTESIAN_POINT ( 'NONE',  ( -37.02382435302582309, -48.24859572486943904, 7.102600956461226467 ) ) ;
#8318=CARTESIAN_POINT ( 'NONE',  ( -23.64089511245930098, -29.75140427513057517, -6.280328284105564762 ) ) ;
#8327=CARTESIAN_POINT ( 'NONE',  ( -23.95213185889994989, -38.49859572486943904, 5.972947139071243861 ) ) ;
#8328=CARTESIAN_POINT ( 'NONE',  ( -39.38303923565386100, -44.70000000000000284, -1.486127417882099788 ) ) ;
#8330=CARTESIAN_POINT ( 'NONE',  ( -25.63988726744978663, -29.60140427513057659, -8.440510857627391061 ) ) ;
#8334=STYLED_ITEM ( 'NONE', ( #6485 ), #7808 ) ;
#8338=CARTESIAN_POINT ( 'NONE',  ( -28.67030704715798350, -34.80000000000000426, 8.395350895058669494 ) ) ;
#8339=CARTESIAN_POINT ( 'NONE',  ( -21.59636165304264921, -32.19859572486942767, 1.277368040863740228 ) ) ;
#8347=SURFACE_SIDE_STYLE ('',( #4865 ) ) ;
#8348=CARTESIAN_POINT ( 'NONE',  ( -23.98959235991431171, -37.50000000000000711, 6.010407640085604797 ) ) ;
#8353=CARTESIAN_POINT ( 'NONE',  ( -21.09983283352784156, -37.35000000000000853, 4.534861676072186043 ) ) ;
#8355=CARTESIAN_POINT ( 'NONE',  ( -38.46456197978948666, -44.40000000000000568, 4.312909747525784709 ) ) ;
#8361=CARTESIAN_POINT ( 'NONE',  ( -28.61798213517984024, -41.79859572486943620, 8.387063443159973986 ) ) ;
#8362=CARTESIAN_POINT ( 'NONE',  ( -36.75497492228666374, -45.99859572486943904, -6.680053920257780220 ) ) ;
#8363=CARTESIAN_POINT ( 'NONE',  ( -38.48861310195163554, -46.40140427513058086, 4.265706762501153548 ) ) ;
#8367=CARTESIAN_POINT ( 'NONE',  ( -31.56260684030781505, -31.95000000000000639, 9.865911304835510265 ) ) ;
#8373=CARTESIAN_POINT ( 'NONE',  ( -38.81868038277247734, -39.54859572486944330, 1.453139578080855365 ) ) ;
#8376=CARTESIAN_POINT ( 'NONE',  ( -28.51387258211773812, -40.80000000000000426, 9.383039235653802379 ) ) ;
#8379=CARTESIAN_POINT ( 'NONE',  ( -25.68709025247441602, -45.60000000000000853, -8.464561979789547053 ) ) ;
#8386=CARTESIAN_POINT ( 'NONE',  ( -38.82739432537914581, -32.55000000000000426, 1.398121909749243441 ) ) ;
#8393=CARTESIAN_POINT ( 'NONE',  ( -28.67030704715798350, -37.80000000000000426, 8.395350895058669494 ) ) ;
#8398=CARTESIAN_POINT ( 'NONE',  ( -37.06321265474346660, -35.24999999999998579, 7.063212654743582952 ) ) ;
#8400=CARTESIAN_POINT ( 'NONE',  ( -39.86591130483550671, -41.55000000000000426, 1.562606840307984690 ) ) ;
#8401=FILL_AREA_STYLE ('',( #5041 ) ) ;
#8404=CARTESIAN_POINT ( 'NONE',  ( -22.45049566656107842, -37.89859572486944472, -3.906122232810846917 ) ) ;
#8405=CARTESIAN_POINT ( 'NONE',  ( -20.60867331244750034, -50.19859572486944188, 1.433802505903951419 ) ) ;
#8406=CARTESIAN_POINT ( 'NONE',  ( -21.16389173201424612, -33.05140427513057233, -1.343104241417630185 ) ) ;
#8410=CARTESIAN_POINT ( 'NONE',  ( -39.38303923565386100, -38.70000000000000284, -1.486127417882099788 ) ) ;
#8417=CARTESIAN_POINT ( 'NONE',  ( -38.81868038277247734, -42.54859572486944330, 1.453139578080855365 ) ) ;
#8418=CARTESIAN_POINT ( 'NONE',  ( -31.48612741788231517, -42.30000000000000426, -9.383039235653804155 ) ) ;
#8421=CARTESIAN_POINT ( 'NONE',  ( -21.12512167993187973, -33.35140427513057659, 4.584493831696868860 ) ) ;
#8428=CARTESIAN_POINT ( 'NONE',  ( -31.32969295284206979, -36.30000000000000426, -8.395350895058669494 ) ) ;
#8431=CARTESIAN_POINT ( 'NONE',  ( -36.31971658582311591, -50.24999999999999289, 6.319716585823200283 ) ) ;
#8435=CARTESIAN_POINT ( 'NONE',  ( -33.85891924778610473, -44.10000000000000853, 7.573555455601171715 ) ) ;
#8438=CARTESIAN_POINT ( 'NONE',  ( -31.32969295284206979, -30.30000000000000782, -8.395350895058669494 ) ) ;
#8439=CARTESIAN_POINT ( 'NONE',  ( -38.46456197978948666, -32.40000000000000568, 4.312909747525784709 ) ) ;
#8441=CARTESIAN_POINT ( 'NONE',  ( -28.43739315969223824, -36.44999999999999574, -9.865911304835512041 ) ) ;
#8445=CARTESIAN_POINT ( 'NONE',  ( -31.53845232986046554, -31.29859572486943975, -9.374751783755117529 ) ) ;
#8446=CARTESIAN_POINT ( 'NONE',  ( -22.97617564697422665, -49.74859572486944614, -7.102600956461224690 ) ) ;
#8447=CARTESIAN_POINT ( 'NONE',  ( -31.27736804086391942, -38.30140427513057944, -8.403638346957361449 ) ) ;
#8451=CARTESIAN_POINT ( 'NONE',  ( -39.86591130483550671, -35.55000000000001137, 1.562606840307984468 ) ) ;
#8457=CARTESIAN_POINT ( 'NONE',  ( -31.34310424141748896, -38.94859572486943478, 8.836108267985801845 ) ) ;
#8458=CARTESIAN_POINT ( 'NONE',  ( -34.53486167607238144, -45.14999999999999858, -8.900167166472096270 ) ) ;
#8460=CARTESIAN_POINT ( 'NONE',  ( -39.37475178375516549, -34.70140427513057091, -1.538452329860249712 ) ) ;
#8469=CARTESIAN_POINT ( 'NONE',  ( -28.60187809025093841, -33.45000000000000995, -8.827394325379140483 ) ) ;
#8480=CARTESIAN_POINT ( 'NONE',  ( -31.48612741788231517, -36.30000000000000426, -9.383039235653804155 ) ) ;
#8482=CARTESIAN_POINT ( 'NONE',  ( -28.65689575858256077, -46.44859572486943478, -8.836108267985801845 ) ) ;
#8483=CARTESIAN_POINT ( 'NONE',  ( -34.31290974752564438, -41.10000000000000142, 8.464561979789547053 ) ) ;
#8485=CARTESIAN_POINT ( 'NONE',  ( -22.40239342223677355, -38.90140427513058086, -3.811716262761597473 ) ) ;
#8488=CARTESIAN_POINT ( 'NONE',  ( -20.61696076434619584, -34.20000000000000995, 1.486127417882100676 ) ) ;
#8497=CARTESIAN_POINT ( 'NONE',  ( -39.85719736222883824, -33.54859572486944330, 1.617624508639602388 ) ) ;
#8498=CARTESIAN_POINT ( 'NONE',  ( -20.62524821624488069, -30.20140427513057446, 1.538452329860250378 ) ) ;
#8501=CARTESIAN_POINT ( 'NONE',  ( -39.87462524744216807, -40.55140427513058654, 1.507589171976367215 ) ) ;
#8508=CARTESIAN_POINT ( 'NONE',  ( -24.02705286092866643, -48.50140427513058938, 6.047868141099968398 ) ) ;
#8519=CARTESIAN_POINT ( 'NONE',  ( -28.51387258211773812, -49.80000000000001137, 9.383039235653802379 ) ) ;
#8521=CARTESIAN_POINT ( 'NONE',  ( -20.14280263777121149, -32.04859572486944330, -1.617624508639600833 ) ) ;
#8522=CARTESIAN_POINT ( 'NONE',  ( -20.13408869516453947, -37.05000000000001137, -1.562606840307983136 ) ) ;
#8523=CARTESIAN_POINT ( 'NONE',  ( -38.38706344316003793, -37.70140427513057091, -1.382017864820032083 ) ) ;
#8527=CARTESIAN_POINT ( 'NONE',  ( -31.50758917197619979, -35.94859572486944188, 9.874625247442176956 ) ) ;
#8528=CARTESIAN_POINT ( 'NONE',  ( -36.71751442127229836, -33.00000000000000711, -6.717514421272142044 ) ) ;
#8536=CARTESIAN_POINT ( 'NONE',  ( -36.04786814110010340, -51.99859572486943193, -5.972947139071243861 ) ) ;
#8537=CARTESIAN_POINT ( 'NONE',  ( -38.48861310195163554, -34.40140427513058086, 4.265706762501153548 ) ) ;
#8540=CARTESIAN_POINT ( 'NONE',  ( -34.36011273255026310, -37.10140427513057659, 8.440510857627391061 ) ) ;
#8548=CARTESIAN_POINT ( 'NONE',  ( -38.82739432537914581, -44.55000000000001137, 1.398121909749243441 ) ) ;
#8556=CARTESIAN_POINT ( 'NONE',  ( -21.16389173201424612, -36.05140427513057944, -1.343104241417630185 ) ) ;
#8560=CARTESIAN_POINT ( 'NONE',  ( -21.60464910494133406, -37.20000000000000284, 1.329692952841886155 ) ) ;
#8565=CARTESIAN_POINT ( 'NONE',  ( -38.81868038277247734, -48.54859572486944330, 1.453139578080855365 ) ) ;
#8566=CARTESIAN_POINT ( 'NONE',  ( -23.28248557872775137, -40.50000000000000711, 6.717514421272141156 ) ) ;
#8567=CARTESIAN_POINT ( 'NONE',  ( -22.06198138166579170, -36.35140427513057659, 4.107139971057695682 ) ) ;
#8570=CARTESIAN_POINT ( 'NONE',  ( -21.07454398712378918, -41.34859572486944757, 4.485229520447505003 ) ) ;
#8571=CARTESIAN_POINT ( 'NONE',  ( -31.56260684030781505, -34.95000000000000995, 9.865911304835510265 ) ) ;
#8577=CARTESIAN_POINT ( 'NONE',  ( -31.53845232986046554, -34.29859572486943620, -9.374751783755117529 ) ) ;
#8578=CARTESIAN_POINT ( 'NONE',  ( -28.51387258211773812, -49.80000000000001137, 9.383039235653802379 ) ) ;
#8581=CARTESIAN_POINT ( 'NONE',  ( -21.12512167993187973, -36.35140427513057659, 4.584493831696868860 ) ) ;
#8588=CARTESIAN_POINT ( 'NONE',  ( -36.31971658582311591, -44.25000000000000000, 6.319716585823199395 ) ) ;
#8595=CARTESIAN_POINT ( 'NONE',  ( -20.61696076434619584, -40.20000000000000995, 1.486127417882100676 ) ) ;
#8598=CARTESIAN_POINT ( 'NONE',  ( -36.35910488754074521, -31.25140427513058228, 6.280328284105565650 ) ) ;
#8602=CARTESIAN_POINT ( 'NONE',  ( -34.05750781543319050, -36.15000000000000568, -7.963307464738194952 ) ) ;
#8604=CARTESIAN_POINT ( 'NONE',  ( -22.93678734525658314, -48.75000000000000711, -7.063212654743582064 ) ) ;
#8607=CARTESIAN_POINT ( 'NONE',  ( -36.28032828410546529, -51.24859572486943193, 6.359104887540839357 ) ) ;
#8608=CARTESIAN_POINT ( 'NONE',  ( -38.46456197978948666, -35.40000000000000568, 4.312909747525784709 ) ) ;
#8609=CARTESIAN_POINT ( 'NONE',  ( -22.40239342223677355, -41.90140427513058086, -3.811716262761597473 ) ) ;
#8614=CARTESIAN_POINT ( 'NONE',  ( -37.02382435302582309, -42.24859572486943904, 7.102600956461226467 ) ) ;
#8615=CARTESIAN_POINT ( 'NONE',  ( -28.43739315969223824, -42.44999999999999574, -9.865911304835512041 ) ) ;
#8623=CARTESIAN_POINT ( 'NONE',  ( -36.28032828410546529, -51.24859572486943193, 6.359104887540839357 ) ) ;
#8624=CARTESIAN_POINT ( 'NONE',  ( -25.63988726744978663, -35.60140427513057659, -8.440510857627391061 ) ) ;
#8628=CARTESIAN_POINT ( 'NONE',  ( -28.38237549136062654, -47.45140427513057091, -9.857197362228843573 ) ) ;
#8636=CARTESIAN_POINT ( 'NONE',  ( -34.05750781543318340, -39.14999999999999147, -7.963307464738195840 ) ) ;
#8641=CARTESIAN_POINT ( 'NONE',  ( -39.38303923565386100, -44.70000000000000284, -1.486127417882099788 ) ) ;
#8644=CARTESIAN_POINT ( 'NONE',  ( -28.54686042191934092, -38.45140427513057801, -8.818680382772479120 ) ) ;
#8647=CARTESIAN_POINT ( 'NONE',  ( -21.17260567462091103, -40.05000000000001137, -1.398121909749241887 ) ) ;
#8650=CARTESIAN_POINT ( 'NONE',  ( -25.68709025247441602, -45.60000000000000853, -8.464561979789547053 ) ) ;
#8652=VERTEX_POINT ( 'NONE', #3778 ) ;
#8654=CARTESIAN_POINT ( 'NONE',  ( -38.90016716647221529, -35.84999999999998721, -4.534861676072185155 ) ) ;
#8655=CARTESIAN_POINT ( 'NONE',  ( -31.39812190974910422, -31.95000000000000639, 8.827394325379140483 ) ) ;
#8658=CARTESIAN_POINT ( 'NONE',  ( -36.75497492228666374, -33.99859572486943904, -6.680053920257780220 ) ) ;
#8664=CARTESIAN_POINT ( 'NONE',  ( -21.18131961722757595, -32.04859572486944330, -1.453139578080854699 ) ) ;
#8665=CARTESIAN_POINT ( 'NONE',  ( -39.39132668755255651, -33.69859572486942767, -1.433802505903950308 ) ) ;
#8666=CARTESIAN_POINT ( 'NONE',  ( -21.12512167993187973, -36.35140427513057659, 4.584493831696868860 ) ) ;
#8669=CARTESIAN_POINT ( 'NONE',  ( -35.97294713907137975, -29.00140427513058583, -6.047868141099968398 ) ) ;
#8676=CARTESIAN_POINT ( 'NONE',  ( -22.42644454439892598, -45.90000000000001279, -3.858919247786222861 ) ) ;
#8680=CARTESIAN_POINT ( 'NONE',  ( -37.06321265474346660, -47.25000000000000711, 7.063212654743582952 ) ) ;
#8683=CARTESIAN_POINT ( 'NONE',  ( -26.09387776718931917, -38.60140427513057659, -7.549504333439021941 ) ) ;
#8686=CARTESIAN_POINT ( 'NONE',  ( -21.60464910494133406, -34.20000000000000995, 1.329692952841886155 ) ) ;
#8688=CARTESIAN_POINT ( 'NONE',  ( -21.53543802021056663, -45.90000000000001279, -4.312909747525783821 ) ) ;
#8692=CARTESIAN_POINT ( 'NONE',  ( -28.51387258211773812, -43.80000000000000426, 9.383039235653802379 ) ) ;
#8693=CARTESIAN_POINT ( 'NONE',  ( -22.06198138166579170, -48.35140427513057659, 4.107139971057695682 ) ) ;
#8696=CARTESIAN_POINT ( 'NONE',  ( -20.14280263777121149, -38.04859572486944330, -1.617624508639600833 ) ) ;
#8703=CARTESIAN_POINT ( 'NONE',  ( -21.59636165304264921, -32.19859572486942767, 1.277368040863740228 ) ) ;
#8704=CARTESIAN_POINT ( 'NONE',  ( -28.46154767013959486, -35.79859572486943620, 9.374751783755112200 ) ) ;
#8705=CARTESIAN_POINT ( 'NONE',  ( -21.51138689804841420, -44.90140427513058086, -4.265706762501151772 ) ) ;
#8709=CARTESIAN_POINT ( 'NONE',  ( -38.48861310195163554, -49.40140427513058086, 4.265706762501153548 ) ) ;
ENDSEC;
END-ISO-10303-21;
